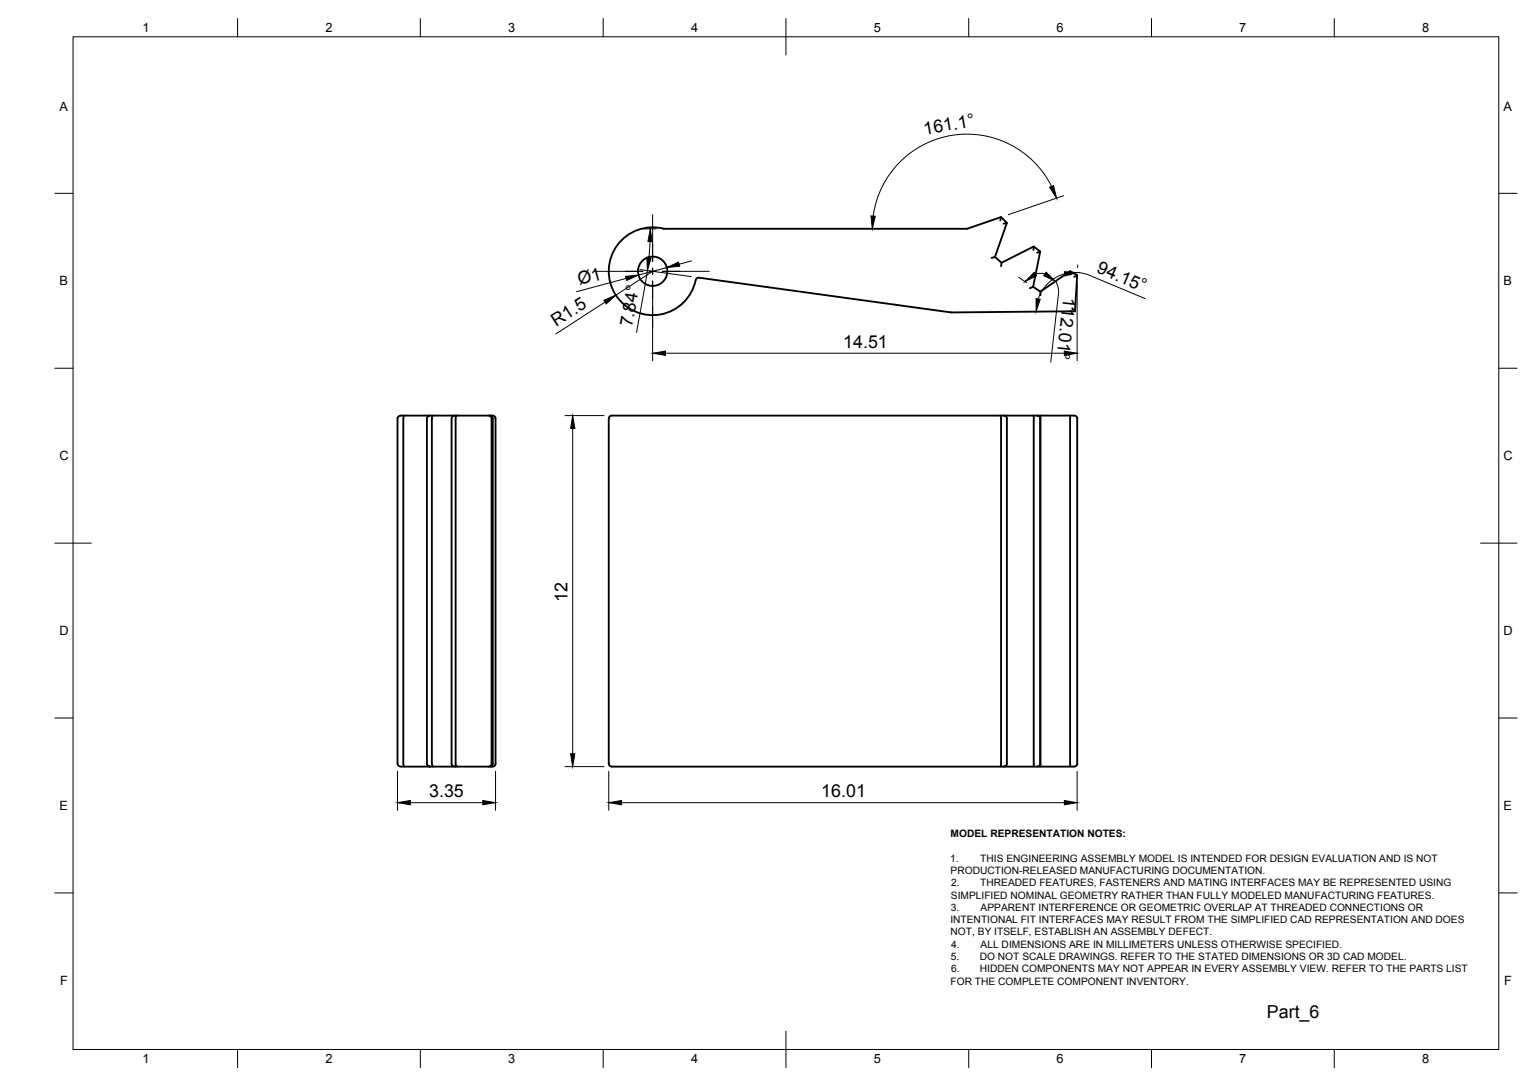
ISO-10303-21;
HEADER;
/* Generated by software containing ST-Developer
 * from STEP Tools, Inc. (www.steptools.com) 
 */

FILE_DESCRIPTION(
/* description */ ('STEP AP242 Edition 2'),
/* implementation_level */ '2;1');

FILE_NAME(
/* name */ 'Part_6.step',
/* time_stamp */ '2026-10-06T10:11:12-07:00',
/* author */ (''),
/* organization */ (''),
/* preprocessor_version */ 'ST-DEVELOPER v20.2',
/* originating_system */ 'Autodesk Translation Framework v15.15.0.0',
/* authorisation */ '');

FILE_SCHEMA (('AUTOMOTIVE_DESIGN { 1 0 10303 214 3 1 1 }'));
ENDSEC;

DATA;
#10=MECHANICAL_DESIGN_GEOMETRIC_PRESENTATION_REPRESENTATION('',(#1793),#54580);
#98=ELLIPSE('',#18957,0.000117970312899575,0.0001);
#99=ELLIPSE('',#18958,0.000120617936713865,0.0001);
#100=ELLIPSE('',#18960,0.000120617936713866,0.0001);
#101=ELLIPSE('',#18962,0.000120617936713866,0.0001);
#102=ELLIPSE('',#18963,0.000120617936713865,0.0001);
#103=ELLIPSE('',#18965,0.000117970312899575,0.0001);
#104=ELLIPSE('',#18967,0.000117970312899575,0.0001);
#105=ELLIPSE('',#18969,0.000117970312899574,0.0001);
#106=ELLIPSE('',#18971,0.000117970312899574,0.0001);
#107=ELLIPSE('',#18973,0.000117970312899575,0.0001);
#108=ELLIPSE('',#18975,0.000120617936713865,0.0001);
#109=ELLIPSE('',#18977,0.000117970312899575,0.0001);
#110=ELLIPSE('',#18979,0.000117970312899575,0.0001);
#111=ELLIPSE('',#18981,0.000120617936713865,0.0001);
#112=ELLIPSE('',#18983,0.000120617936713865,0.0001);
#113=ELLIPSE('',#18985,0.000136567519156022,0.0001);
#114=ELLIPSE('',#18987,0.000136567519156022,0.0001);
#115=ELLIPSE('',#18989,0.000120617936713865,0.0001);
#116=ELLIPSE('',#18991,0.000117970312899574,0.0001);
#117=ELLIPSE('',#19000,0.000117970312899574,0.0001);
#118=ELLIPSE('',#19002,0.000117970312899575,0.0001);
#119=ELLIPSE('',#19008,0.000117970312899575,0.0001);
#149=SPHERICAL_SURFACE('',#19003,0.0001);
#150=SPHERICAL_SURFACE('',#19005,0.0001);
#248=TOROIDAL_SURFACE('',#19023,0.0002,0.0001);
#249=TOROIDAL_SURFACE('',#19025,0.0002,0.0001);
#250=TOROIDAL_SURFACE('',#19027,0.0002,0.0001);
#251=TOROIDAL_SURFACE('',#19029,0.0002,0.0001);
#252=TOROIDAL_SURFACE('',#19033,0.0014,0.0001);
#253=TOROIDAL_SURFACE('',#19035,0.0014,0.0001);
#254=TOROIDAL_SURFACE('',#19039,0.0002,0.0001);
#255=TOROIDAL_SURFACE('',#19041,0.0002,0.0001);
#256=TOROIDAL_SURFACE('',#19044,0.0006,0.0001);
#257=TOROIDAL_SURFACE('',#19046,0.0006,0.0001);
#1749=SHAPE_REPRESENTATION_RELATIONSHIP('SRR','None',#54636,#1763);
#1763=ADVANCED_BREP_SHAPE_REPRESENTATION('',(#1807),#54572);
#1793=STYLED_ITEM('',(#54717),#1807);
#1807=MANIFOLD_SOLID_BREP('Body1',#17672);
#2175=LINE('',#48245,#2768);
#2176=LINE('',#48249,#2769);
#2177=LINE('',#48254,#2770);
#2178=LINE('',#48256,#2771);
#2179=LINE('',#48258,#2772);
#2180=LINE('',#48259,#2773);
#2181=LINE('',#48263,#2774);
#2182=LINE('',#48265,#2775);
#2183=LINE('',#48267,#2776);
#2184=LINE('',#48268,#2777);
#2185=LINE('',#48272,#2778);
#2186=LINE('',#48273,#2779);
#2187=LINE('',#48274,#2780);
#2188=LINE('',#48278,#2781);
#2189=LINE('',#48279,#2782);
#2190=LINE('',#48280,#2783);
#2191=LINE('',#48284,#2784);
#2192=LINE('',#48285,#2785);
#2193=LINE('',#48286,#2786);
#2194=LINE('',#48290,#2787);
#2195=LINE('',#48291,#2788);
#2196=LINE('',#48292,#2789);
#2197=LINE('',#48296,#2790);
#2198=LINE('',#48297,#2791);
#2199=LINE('',#48298,#2792);
#2200=LINE('',#48302,#2793);
#2201=LINE('',#48303,#2794);
#2202=LINE('',#48304,#2795);
#2203=LINE('',#48308,#2796);
#2204=LINE('',#48309,#2797);
#2205=LINE('',#48310,#2798);
#2206=LINE('',#48314,#2799);
#2207=LINE('',#48315,#2800);
#2208=LINE('',#48316,#2801);
#2209=LINE('',#48320,#2802);
#2210=LINE('',#48321,#2803);
#2211=LINE('',#48322,#2804);
#2212=LINE('',#48326,#2805);
#2213=LINE('',#48327,#2806);
#2214=LINE('',#48328,#2807);
#2215=LINE('',#48332,#2808);
#2216=LINE('',#48333,#2809);
#2217=LINE('',#48334,#2810);
#2218=LINE('',#48338,#2811);
#2219=LINE('',#48340,#2812);
#2220=LINE('',#48342,#2813);
#2221=LINE('',#48343,#2814);
#2222=LINE('',#48347,#2815);
#2223=LINE('',#48349,#2816);
#2224=LINE('',#48351,#2817);
#2225=LINE('',#48359,#2818);
#2226=LINE('',#48363,#2819);
#2227=LINE('',#48365,#2820);
#2228=LINE('',#48367,#2821);
#2229=LINE('',#48369,#2822);
#2230=LINE('',#48371,#2823);
#2231=LINE('',#48373,#2824);
#2232=LINE('',#48375,#2825);
#2233=LINE('',#48377,#2826);
#2234=LINE('',#48379,#2827);
#2235=LINE('',#48380,#2828);
#2236=LINE('',#48386,#2829);
#2237=LINE('',#48388,#2830);
#2238=LINE('',#48390,#2831);
#2239=LINE('',#48394,#2832);
#2240=LINE('',#48402,#2833);
#2241=LINE('',#48404,#2834);
#2242=LINE('',#48406,#2835);
#2243=LINE('',#48408,#2836);
#2244=LINE('',#48410,#2837);
#2245=LINE('',#48412,#2838);
#2246=LINE('',#48414,#2839);
#2247=LINE('',#48416,#2840);
#2248=LINE('',#48418,#2841);
#2249=LINE('',#48419,#2842);
#2250=LINE('',#48428,#2843);
#2768=VECTOR('',#22139,1.);
#2769=VECTOR('',#22142,1.);
#2770=VECTOR('',#22147,1.);
#2771=VECTOR('',#22148,1.);
#2772=VECTOR('',#22149,1.);
#2773=VECTOR('',#22150,1.);
#2774=VECTOR('',#22153,1.);
#2775=VECTOR('',#22154,1.);
#2776=VECTOR('',#22155,1.);
#2777=VECTOR('',#22156,1.);
#2778=VECTOR('',#22159,1.);
#2779=VECTOR('',#22160,1.);
#2780=VECTOR('',#22161,1.);
#2781=VECTOR('',#22164,1.);
#2782=VECTOR('',#22165,1.);
#2783=VECTOR('',#22166,1.);
#2784=VECTOR('',#22169,1.);
#2785=VECTOR('',#22170,1.);
#2786=VECTOR('',#22171,1.);
#2787=VECTOR('',#22174,1.);
#2788=VECTOR('',#22175,0.999999999999999);
#2789=VECTOR('',#22176,0.999999999999999);
#2790=VECTOR('',#22179,1.);
#2791=VECTOR('',#22180,1.);
#2792=VECTOR('',#22181,1.);
#2793=VECTOR('',#22184,1.);
#2794=VECTOR('',#22185,1.);
#2795=VECTOR('',#22186,1.);
#2796=VECTOR('',#22189,1.);
#2797=VECTOR('',#22190,1.);
#2798=VECTOR('',#22191,1.);
#2799=VECTOR('',#22194,1.);
#2800=VECTOR('',#22195,1.);
#2801=VECTOR('',#22196,1.);
#2802=VECTOR('',#22199,1.);
#2803=VECTOR('',#22200,1.);
#2804=VECTOR('',#22201,1.);
#2805=VECTOR('',#22204,1.);
#2806=VECTOR('',#22205,1.);
#2807=VECTOR('',#22206,1.);
#2808=VECTOR('',#22209,1.);
#2809=VECTOR('',#22210,1.);
#2810=VECTOR('',#22211,1.);
#2811=VECTOR('',#22214,1.);
#2812=VECTOR('',#22215,1.);
#2813=VECTOR('',#22216,1.);
#2814=VECTOR('',#22217,1.);
#2815=VECTOR('',#22220,1.);
#2816=VECTOR('',#22221,1.);
#2817=VECTOR('',#22222,1.);
#2818=VECTOR('',#22229,1.);
#2819=VECTOR('',#22232,1.);
#2820=VECTOR('',#22233,1.);
#2821=VECTOR('',#22234,1.);
#2822=VECTOR('',#22235,1.);
#2823=VECTOR('',#22236,1.);
#2824=VECTOR('',#22237,1.);
#2825=VECTOR('',#22238,1.);
#2826=VECTOR('',#22239,0.999999999999999);
#2827=VECTOR('',#22240,1.);
#2828=VECTOR('',#22241,1.);
#2829=VECTOR('',#22246,1.);
#2830=VECTOR('',#22247,1.);
#2831=VECTOR('',#22248,1.);
#2832=VECTOR('',#22251,1.);
#2833=VECTOR('',#22258,1.);
#2834=VECTOR('',#22259,1.);
#2835=VECTOR('',#22260,1.);
#2836=VECTOR('',#22261,1.);
#2837=VECTOR('',#22262,1.);
#2838=VECTOR('',#22263,0.999999999999999);
#2839=VECTOR('',#22264,1.);
#2840=VECTOR('',#22265,1.);
#2841=VECTOR('',#22266,1.);
#2842=VECTOR('',#22267,1.);
#2843=VECTOR('',#22276,0.0005);
#3361=CYLINDRICAL_SURFACE('',#18923,0.0015);
#3362=CYLINDRICAL_SURFACE('',#18952,0.0005);
#3363=CYLINDRICAL_SURFACE('',#18956,0.0001);
#3364=CYLINDRICAL_SURFACE('',#18959,0.0001);
#3365=CYLINDRICAL_SURFACE('',#18961,0.0001);
#3366=CYLINDRICAL_SURFACE('',#18964,0.0001);
#3367=CYLINDRICAL_SURFACE('',#18966,0.0001);
#3368=CYLINDRICAL_SURFACE('',#18968,0.0001);
#3369=CYLINDRICAL_SURFACE('',#18970,0.0001);
#3370=CYLINDRICAL_SURFACE('',#18972,0.0001);
#3371=CYLINDRICAL_SURFACE('',#18974,0.0001);
#3372=CYLINDRICAL_SURFACE('',#18976,0.0001);
#3373=CYLINDRICAL_SURFACE('',#18978,0.0001);
#3374=CYLINDRICAL_SURFACE('',#18980,0.0001);
#3375=CYLINDRICAL_SURFACE('',#18982,0.0001);
#3376=CYLINDRICAL_SURFACE('',#18984,0.0001);
#3377=CYLINDRICAL_SURFACE('',#18986,0.0001);
#3378=CYLINDRICAL_SURFACE('',#18988,0.0001);
#3379=CYLINDRICAL_SURFACE('',#18990,0.0001);
#3380=CYLINDRICAL_SURFACE('',#18992,0.0001);
#3381=CYLINDRICAL_SURFACE('',#18994,0.0001);
#3382=CYLINDRICAL_SURFACE('',#18997,0.0001);
#3383=CYLINDRICAL_SURFACE('',#18999,0.0001);
#3384=CYLINDRICAL_SURFACE('',#19001,0.0001);
#3385=CYLINDRICAL_SURFACE('',#19007,0.0001);
#3386=CYLINDRICAL_SURFACE('',#19009,0.0001);
#3387=CYLINDRICAL_SURFACE('',#19011,0.0001);
#3388=CYLINDRICAL_SURFACE('',#19013,0.0001);
#3389=CYLINDRICAL_SURFACE('',#19016,0.0001);
#3390=CYLINDRICAL_SURFACE('',#19018,0.0001);
#3391=CYLINDRICAL_SURFACE('',#19020,0.0001);
#3392=CYLINDRICAL_SURFACE('',#19031,0.0001);
#3393=CYLINDRICAL_SURFACE('',#19037,0.0001);
#3394=CYLINDRICAL_SURFACE('',#19043,0.0001);
#3508=FACE_BOUND('',#5278,.T.);
#3509=FACE_BOUND('',#5280,.T.);
#4225=FACE_OUTER_BOUND('',#5262,.T.);
#4226=FACE_OUTER_BOUND('',#5263,.T.);
#4227=FACE_OUTER_BOUND('',#5264,.T.);
#4228=FACE_OUTER_BOUND('',#5265,.T.);
#4229=FACE_OUTER_BOUND('',#5266,.T.);
#4230=FACE_OUTER_BOUND('',#5267,.T.);
#4231=FACE_OUTER_BOUND('',#5268,.T.);
#4232=FACE_OUTER_BOUND('',#5269,.T.);
#4233=FACE_OUTER_BOUND('',#5270,.T.);
#4234=FACE_OUTER_BOUND('',#5271,.T.);
#4235=FACE_OUTER_BOUND('',#5272,.T.);
#4236=FACE_OUTER_BOUND('',#5273,.T.);
#4237=FACE_OUTER_BOUND('',#5274,.T.);
#4238=FACE_OUTER_BOUND('',#5275,.T.);
#4239=FACE_OUTER_BOUND('',#5276,.T.);
#4240=FACE_OUTER_BOUND('',#5277,.T.);
#4241=FACE_OUTER_BOUND('',#5279,.T.);
#4242=FACE_OUTER_BOUND('',#5281,.T.);
#4243=FACE_OUTER_BOUND('',#5282,.T.);
#4244=FACE_OUTER_BOUND('',#5283,.T.);
#4245=FACE_OUTER_BOUND('',#5284,.T.);
#4246=FACE_OUTER_BOUND('',#5285,.T.);
#4247=FACE_OUTER_BOUND('',#5286,.T.);
#4248=FACE_OUTER_BOUND('',#5287,.T.);
#4249=FACE_OUTER_BOUND('',#5288,.T.);
#4250=FACE_OUTER_BOUND('',#5289,.T.);
#4251=FACE_OUTER_BOUND('',#5290,.T.);
#4252=FACE_OUTER_BOUND('',#5291,.T.);
#4253=FACE_OUTER_BOUND('',#5292,.T.);
#4254=FACE_OUTER_BOUND('',#5293,.T.);
#4255=FACE_OUTER_BOUND('',#5294,.T.);
#4256=FACE_OUTER_BOUND('',#5295,.T.);
#4257=FACE_OUTER_BOUND('',#5296,.T.);
#4258=FACE_OUTER_BOUND('',#5297,.T.);
#4259=FACE_OUTER_BOUND('',#5298,.T.);
#4260=FACE_OUTER_BOUND('',#5299,.T.);
#4261=FACE_OUTER_BOUND('',#5300,.T.);
#4262=FACE_OUTER_BOUND('',#5301,.T.);
#4263=FACE_OUTER_BOUND('',#5302,.T.);
#4264=FACE_OUTER_BOUND('',#5303,.T.);
#4265=FACE_OUTER_BOUND('',#5304,.T.);
#4266=FACE_OUTER_BOUND('',#5305,.T.);
#4267=FACE_OUTER_BOUND('',#5306,.T.);
#4268=FACE_OUTER_BOUND('',#5307,.T.);
#4269=FACE_OUTER_BOUND('',#5308,.T.);
#4270=FACE_OUTER_BOUND('',#5309,.T.);
#4271=FACE_OUTER_BOUND('',#5310,.T.);
#4272=FACE_OUTER_BOUND('',#5311,.T.);
#4273=FACE_OUTER_BOUND('',#5312,.T.);
#4274=FACE_OUTER_BOUND('',#5313,.T.);
#4275=FACE_OUTER_BOUND('',#5314,.T.);
#4276=FACE_OUTER_BOUND('',#5315,.T.);
#4277=FACE_OUTER_BOUND('',#5316,.T.);
#4278=FACE_OUTER_BOUND('',#5317,.T.);
#4279=FACE_OUTER_BOUND('',#5318,.T.);
#4280=FACE_OUTER_BOUND('',#5319,.T.);
#4281=FACE_OUTER_BOUND('',#5320,.T.);
#4282=FACE_OUTER_BOUND('',#5321,.T.);
#4283=FACE_OUTER_BOUND('',#5322,.T.);
#4284=FACE_OUTER_BOUND('',#5323,.T.);
#4285=FACE_OUTER_BOUND('',#5324,.T.);
#4286=FACE_OUTER_BOUND('',#5325,.T.);
#5262=EDGE_LOOP('',(#14995,#14996,#14997,#14998));
#5263=EDGE_LOOP('',(#14999,#15000,#15001,#15002));
#5264=EDGE_LOOP('',(#15003,#15004,#15005,#15006));
#5265=EDGE_LOOP('',(#15007,#15008,#15009,#15010));
#5266=EDGE_LOOP('',(#15011,#15012,#15013,#15014));
#5267=EDGE_LOOP('',(#15015,#15016,#15017,#15018));
#5268=EDGE_LOOP('',(#15019,#15020,#15021,#15022));
#5269=EDGE_LOOP('',(#15023,#15024,#15025,#15026));
#5270=EDGE_LOOP('',(#15027,#15028,#15029,#15030));
#5271=EDGE_LOOP('',(#15031,#15032,#15033,#15034));
#5272=EDGE_LOOP('',(#15035,#15036,#15037,#15038));
#5273=EDGE_LOOP('',(#15039,#15040,#15041,#15042));
#5274=EDGE_LOOP('',(#15043,#15044,#15045,#15046));
#5275=EDGE_LOOP('',(#15047,#15048,#15049,#15050));
#5276=EDGE_LOOP('',(#15051,#15052,#15053,#15054));
#5277=EDGE_LOOP('',(#15055,#15056,#15057,#15058,#15059,#15060,#15061,#15062,
#15063,#15064,#15065,#15066,#15067,#15068,#15069,#15070,#15071,#15072));
#5278=EDGE_LOOP('',(#15073));
#5279=EDGE_LOOP('',(#15074,#15075,#15076,#15077,#15078,#15079,#15080,#15081,
#15082,#15083,#15084,#15085,#15086,#15087,#15088,#15089,#15090,#15091));
#5280=EDGE_LOOP('',(#15092));
#5281=EDGE_LOOP('',(#15093,#15094,#15095,#15096,#15097));
#5282=EDGE_LOOP('',(#15098,#15099,#15100,#15101));
#5283=EDGE_LOOP('',(#15102,#15103,#15104,#15105));
#5284=EDGE_LOOP('',(#15106,#15107,#15108,#15109));
#5285=EDGE_LOOP('',(#15110,#15111,#15112,#15113));
#5286=EDGE_LOOP('',(#15114,#15115,#15116,#15117));
#5287=EDGE_LOOP('',(#15118,#15119,#15120,#15121));
#5288=EDGE_LOOP('',(#15122,#15123,#15124,#15125));
#5289=EDGE_LOOP('',(#15126,#15127,#15128,#15129));
#5290=EDGE_LOOP('',(#15130,#15131,#15132,#15133));
#5291=EDGE_LOOP('',(#15134,#15135,#15136,#15137));
#5292=EDGE_LOOP('',(#15138,#15139,#15140,#15141));
#5293=EDGE_LOOP('',(#15142,#15143,#15144,#15145));
#5294=EDGE_LOOP('',(#15146,#15147,#15148,#15149));
#5295=EDGE_LOOP('',(#15150,#15151,#15152,#15153));
#5296=EDGE_LOOP('',(#15154,#15155,#15156,#15157));
#5297=EDGE_LOOP('',(#15158,#15159,#15160,#15161));
#5298=EDGE_LOOP('',(#15162,#15163,#15164,#15165));
#5299=EDGE_LOOP('',(#15166,#15167,#15168,#15169));
#5300=EDGE_LOOP('',(#15170,#15171,#15172,#15173));
#5301=EDGE_LOOP('',(#15174,#15175,#15176,#15177));
#5302=EDGE_LOOP('',(#15178,#15179,#15180,#15181));
#5303=EDGE_LOOP('',(#15182,#15183,#15184,#15185));
#5304=EDGE_LOOP('',(#15186,#15187,#15188));
#5305=EDGE_LOOP('',(#15189,#15190,#15191));
#5306=EDGE_LOOP('',(#15192,#15193,#15194,#15195));
#5307=EDGE_LOOP('',(#15196,#15197,#15198,#15199));
#5308=EDGE_LOOP('',(#15200,#15201,#15202,#15203));
#5309=EDGE_LOOP('',(#15204,#15205,#15206,#15207));
#5310=EDGE_LOOP('',(#15208,#15209,#15210,#15211));
#5311=EDGE_LOOP('',(#15212,#15213,#15214,#15215));
#5312=EDGE_LOOP('',(#15216,#15217,#15218,#15219));
#5313=EDGE_LOOP('',(#15220,#15221,#15222,#15223));
#5314=EDGE_LOOP('',(#15224,#15225,#15226,#15227));
#5315=EDGE_LOOP('',(#15228,#15229,#15230,#15231));
#5316=EDGE_LOOP('',(#15232,#15233,#15234,#15235));
#5317=EDGE_LOOP('',(#15236,#15237,#15238,#15239));
#5318=EDGE_LOOP('',(#15240,#15241,#15242,#15243));
#5319=EDGE_LOOP('',(#15244,#15245,#15246,#15247));
#5320=EDGE_LOOP('',(#15248,#15249,#15250,#15251));
#5321=EDGE_LOOP('',(#15252,#15253,#15254,#15255));
#5322=EDGE_LOOP('',(#15256,#15257,#15258,#15259));
#5323=EDGE_LOOP('',(#15260,#15261,#15262,#15263));
#5324=EDGE_LOOP('',(#15264,#15265,#15266,#15267));
#5325=EDGE_LOOP('',(#15268,#15269,#15270,#15271,#15272));
#6186=CIRCLE('',#18924,0.0015);
#6187=CIRCLE('',#18925,0.0015);
#6188=CIRCLE('',#18941,0.0002);
#6189=CIRCLE('',#18942,0.0014);
#6190=CIRCLE('',#18943,0.0002);
#6191=CIRCLE('',#18944,0.0002);
#6192=CIRCLE('',#18945,0.0006);
#6193=CIRCLE('',#18947,0.0002);
#6194=CIRCLE('',#18948,0.0002);
#6195=CIRCLE('',#18949,0.0014);
#6196=CIRCLE('',#18950,0.0002);
#6197=CIRCLE('',#18951,0.0006);
#6198=CIRCLE('',#18953,0.0005);
#6199=CIRCLE('',#18954,0.0005);
#6200=CIRCLE('',#18955,0.0005);
#6201=CIRCLE('',#18993,0.0001);
#6202=CIRCLE('',#18995,0.0001);
#6203=CIRCLE('',#18996,0.0001);
#6204=CIRCLE('',#18998,0.0001);
#6205=CIRCLE('',#19004,0.0001);
#6206=CIRCLE('',#19006,0.0001);
#6207=CIRCLE('',#19010,0.0001);
#6208=CIRCLE('',#19012,0.0001);
#6209=CIRCLE('',#19014,0.0001);
#6210=CIRCLE('',#19015,0.0001);
#6211=CIRCLE('',#19017,0.0001);
#6212=CIRCLE('',#19019,0.0001);
#6213=CIRCLE('',#19021,0.0001);
#6214=CIRCLE('',#19022,0.0001);
#6215=CIRCLE('',#19024,0.0001);
#6216=CIRCLE('',#19026,0.0001);
#6217=CIRCLE('',#19028,0.0001);
#6218=CIRCLE('',#19030,0.0001);
#6219=CIRCLE('',#19032,0.0001);
#6220=CIRCLE('',#19034,0.0001);
#6221=CIRCLE('',#19036,0.0001);
#6222=CIRCLE('',#19038,0.0001);
#6223=CIRCLE('',#19040,0.0001);
#6224=CIRCLE('',#19042,0.0001);
#6225=CIRCLE('',#19045,0.0001);
#6226=CIRCLE('',#19047,0.0001);
#7845=VERTEX_POINT('',#48243);
#7846=VERTEX_POINT('',#48244);
#7847=VERTEX_POINT('',#48246);
#7848=VERTEX_POINT('',#48248);
#7849=VERTEX_POINT('',#48252);
#7850=VERTEX_POINT('',#48253);
#7851=VERTEX_POINT('',#48255);
#7852=VERTEX_POINT('',#48257);
#7853=VERTEX_POINT('',#48261);
#7854=VERTEX_POINT('',#48262);
#7855=VERTEX_POINT('',#48264);
#7856=VERTEX_POINT('',#48266);
#7857=VERTEX_POINT('',#48270);
#7858=VERTEX_POINT('',#48271);
#7859=VERTEX_POINT('',#48276);
#7860=VERTEX_POINT('',#48277);
#7861=VERTEX_POINT('',#48282);
#7862=VERTEX_POINT('',#48283);
#7863=VERTEX_POINT('',#48288);
#7864=VERTEX_POINT('',#48289);
#7865=VERTEX_POINT('',#48294);
#7866=VERTEX_POINT('',#48295);
#7867=VERTEX_POINT('',#48300);
#7868=VERTEX_POINT('',#48301);
#7869=VERTEX_POINT('',#48306);
#7870=VERTEX_POINT('',#48307);
#7871=VERTEX_POINT('',#48312);
#7872=VERTEX_POINT('',#48313);
#7873=VERTEX_POINT('',#48318);
#7874=VERTEX_POINT('',#48319);
#7875=VERTEX_POINT('',#48324);
#7876=VERTEX_POINT('',#48325);
#7877=VERTEX_POINT('',#48330);
#7878=VERTEX_POINT('',#48331);
#7879=VERTEX_POINT('',#48336);
#7880=VERTEX_POINT('',#48337);
#7881=VERTEX_POINT('',#48339);
#7882=VERTEX_POINT('',#48341);
#7883=VERTEX_POINT('',#48345);
#7884=VERTEX_POINT('',#48346);
#7885=VERTEX_POINT('',#48348);
#7886=VERTEX_POINT('',#48350);
#7887=VERTEX_POINT('',#48352);
#7888=VERTEX_POINT('',#48354);
#7889=VERTEX_POINT('',#48356);
#7890=VERTEX_POINT('',#48358);
#7891=VERTEX_POINT('',#48360);
#7892=VERTEX_POINT('',#48362);
#7893=VERTEX_POINT('',#48364);
#7894=VERTEX_POINT('',#48366);
#7895=VERTEX_POINT('',#48368);
#7896=VERTEX_POINT('',#48370);
#7897=VERTEX_POINT('',#48372);
#7898=VERTEX_POINT('',#48374);
#7899=VERTEX_POINT('',#48376);
#7900=VERTEX_POINT('',#48378);
#7901=VERTEX_POINT('',#48381);
#7902=VERTEX_POINT('',#48384);
#7903=VERTEX_POINT('',#48385);
#7904=VERTEX_POINT('',#48387);
#7905=VERTEX_POINT('',#48389);
#7906=VERTEX_POINT('',#48391);
#7907=VERTEX_POINT('',#48393);
#7908=VERTEX_POINT('',#48395);
#7909=VERTEX_POINT('',#48397);
#7910=VERTEX_POINT('',#48399);
#7911=VERTEX_POINT('',#48401);
#7912=VERTEX_POINT('',#48403);
#7913=VERTEX_POINT('',#48405);
#7914=VERTEX_POINT('',#48407);
#7915=VERTEX_POINT('',#48409);
#7916=VERTEX_POINT('',#48411);
#7917=VERTEX_POINT('',#48413);
#7918=VERTEX_POINT('',#48415);
#7919=VERTEX_POINT('',#48417);
#7920=VERTEX_POINT('',#48420);
#7921=VERTEX_POINT('',#48423);
#7922=VERTEX_POINT('',#48424);
#7923=VERTEX_POINT('',#48427);
#10289=EDGE_CURVE('',#7845,#7846,#2175,.F.);
#10290=EDGE_CURVE('',#7846,#7847,#6186,.F.);
#10291=EDGE_CURVE('',#7847,#7848,#2176,.T.);
#10292=EDGE_CURVE('',#7848,#7845,#6187,.F.);
#10293=EDGE_CURVE('',#7849,#7850,#2177,.F.);
#10294=EDGE_CURVE('',#7850,#7851,#2178,.F.);
#10295=EDGE_CURVE('',#7851,#7852,#2179,.F.);
#10296=EDGE_CURVE('',#7852,#7849,#2180,.T.);
#10297=EDGE_CURVE('',#7853,#7854,#2181,.T.);
#10298=EDGE_CURVE('',#7853,#7855,#2182,.F.);
#10299=EDGE_CURVE('',#7855,#7856,#2183,.T.);
#10300=EDGE_CURVE('',#7856,#7854,#2184,.T.);
#10301=EDGE_CURVE('',#7857,#7858,#2185,.T.);
#10302=EDGE_CURVE('',#7857,#7853,#2186,.F.);
#10303=EDGE_CURVE('',#7854,#7858,#2187,.T.);
#10304=EDGE_CURVE('',#7859,#7860,#2188,.T.);
#10305=EDGE_CURVE('',#7859,#7857,#2189,.F.);
#10306=EDGE_CURVE('',#7858,#7860,#2190,.T.);
#10307=EDGE_CURVE('',#7861,#7862,#2191,.T.);
#10308=EDGE_CURVE('',#7861,#7859,#2192,.F.);
#10309=EDGE_CURVE('',#7860,#7862,#2193,.T.);
#10310=EDGE_CURVE('',#7863,#7864,#2194,.T.);
#10311=EDGE_CURVE('',#7863,#7861,#2195,.F.);
#10312=EDGE_CURVE('',#7862,#7864,#2196,.T.);
#10313=EDGE_CURVE('',#7865,#7866,#2197,.T.);
#10314=EDGE_CURVE('',#7865,#7863,#2198,.F.);
#10315=EDGE_CURVE('',#7864,#7866,#2199,.T.);
#10316=EDGE_CURVE('',#7867,#7868,#2200,.T.);
#10317=EDGE_CURVE('',#7867,#7865,#2201,.F.);
#10318=EDGE_CURVE('',#7866,#7868,#2202,.T.);
#10319=EDGE_CURVE('',#7869,#7870,#2203,.T.);
#10320=EDGE_CURVE('',#7869,#7867,#2204,.F.);
#10321=EDGE_CURVE('',#7868,#7870,#2205,.T.);
#10322=EDGE_CURVE('',#7871,#7872,#2206,.T.);
#10323=EDGE_CURVE('',#7871,#7869,#2207,.F.);
#10324=EDGE_CURVE('',#7870,#7872,#2208,.T.);
#10325=EDGE_CURVE('',#7873,#7874,#2209,.T.);
#10326=EDGE_CURVE('',#7873,#7871,#2210,.F.);
#10327=EDGE_CURVE('',#7872,#7874,#2211,.T.);
#10328=EDGE_CURVE('',#7875,#7876,#2212,.T.);
#10329=EDGE_CURVE('',#7875,#7873,#2213,.F.);
#10330=EDGE_CURVE('',#7874,#7876,#2214,.T.);
#10331=EDGE_CURVE('',#7877,#7878,#2215,.F.);
#10332=EDGE_CURVE('',#7878,#7875,#2216,.F.);
#10333=EDGE_CURVE('',#7876,#7877,#2217,.T.);
#10334=EDGE_CURVE('',#7879,#7880,#2218,.T.);
#10335=EDGE_CURVE('',#7880,#7881,#2219,.F.);
#10336=EDGE_CURVE('',#7881,#7882,#2220,.T.);
#10337=EDGE_CURVE('',#7882,#7879,#2221,.T.);
#10338=EDGE_CURVE('',#7883,#7884,#2222,.F.);
#10339=EDGE_CURVE('',#7884,#7885,#2223,.F.);
#10340=EDGE_CURVE('',#7885,#7886,#2224,.F.);
#10341=EDGE_CURVE('',#7887,#7886,#6188,.T.);
#10342=EDGE_CURVE('',#7887,#7888,#6189,.T.);
#10343=EDGE_CURVE('',#7889,#7888,#6190,.T.);
#10344=EDGE_CURVE('',#7889,#7890,#2225,.F.);
#10345=EDGE_CURVE('',#7891,#7890,#6191,.T.);
#10346=EDGE_CURVE('',#7891,#7892,#2226,.F.);
#10347=EDGE_CURVE('',#7892,#7893,#2227,.F.);
#10348=EDGE_CURVE('',#7893,#7894,#2228,.F.);
#10349=EDGE_CURVE('',#7894,#7895,#2229,.F.);
#10350=EDGE_CURVE('',#7895,#7896,#2230,.F.);
#10351=EDGE_CURVE('',#7896,#7897,#2231,.F.);
#10352=EDGE_CURVE('',#7897,#7898,#2232,.F.);
#10353=EDGE_CURVE('',#7898,#7899,#2233,.F.);
#10354=EDGE_CURVE('',#7899,#7900,#2234,.F.);
#10355=EDGE_CURVE('',#7900,#7883,#2235,.F.);
#10356=EDGE_CURVE('',#7901,#7901,#6192,.F.);
#10357=EDGE_CURVE('',#7902,#7903,#2236,.T.);
#10358=EDGE_CURVE('',#7903,#7904,#2237,.T.);
#10359=EDGE_CURVE('',#7904,#7905,#2238,.T.);
#10360=EDGE_CURVE('',#7906,#7905,#6193,.T.);
#10361=EDGE_CURVE('',#7906,#7907,#2239,.T.);
#10362=EDGE_CURVE('',#7908,#7907,#6194,.T.);
#10363=EDGE_CURVE('',#7908,#7909,#6195,.T.);
#10364=EDGE_CURVE('',#7910,#7909,#6196,.T.);
#10365=EDGE_CURVE('',#7910,#7911,#2240,.T.);
#10366=EDGE_CURVE('',#7911,#7912,#2241,.T.);
#10367=EDGE_CURVE('',#7912,#7913,#2242,.T.);
#10368=EDGE_CURVE('',#7913,#7914,#2243,.T.);
#10369=EDGE_CURVE('',#7914,#7915,#2244,.T.);
#10370=EDGE_CURVE('',#7915,#7916,#2245,.T.);
#10371=EDGE_CURVE('',#7916,#7917,#2246,.T.);
#10372=EDGE_CURVE('',#7917,#7918,#2247,.T.);
#10373=EDGE_CURVE('',#7918,#7919,#2248,.T.);
#10374=EDGE_CURVE('',#7919,#7902,#2249,.T.);
#10375=EDGE_CURVE('',#7920,#7920,#6197,.F.);
#10376=EDGE_CURVE('',#7921,#7922,#6198,.T.);
#10377=EDGE_CURVE('',#7922,#7921,#6199,.T.);
#10378=EDGE_CURVE('',#7921,#7923,#2250,.T.);
#10379=EDGE_CURVE('',#7923,#7923,#6200,.T.);
#10380=EDGE_CURVE('',#7917,#7865,#98,.F.);
#10381=EDGE_CURVE('',#7863,#7916,#99,.T.);
#10382=EDGE_CURVE('',#7861,#7915,#100,.T.);
#10383=EDGE_CURVE('',#7899,#7862,#101,.T.);
#10384=EDGE_CURVE('',#7864,#7898,#102,.F.);
#10385=EDGE_CURVE('',#7866,#7897,#103,.F.);
#10386=EDGE_CURVE('',#7918,#7867,#104,.F.);
#10387=EDGE_CURVE('',#7859,#7914,#105,.T.);
#10388=EDGE_CURVE('',#7900,#7860,#106,.T.);
#10389=EDGE_CURVE('',#7868,#7896,#107,.F.);
#10390=EDGE_CURVE('',#7919,#7869,#108,.F.);
#10391=EDGE_CURVE('',#7857,#7913,#109,.T.);
#10392=EDGE_CURVE('',#7883,#7858,#110,.T.);
#10393=EDGE_CURVE('',#7870,#7895,#111,.F.);
#10394=EDGE_CURVE('',#7902,#7871,#112,.F.);
#10395=EDGE_CURVE('',#7853,#7912,#113,.T.);
#10396=EDGE_CURVE('',#7884,#7854,#114,.T.);
#10397=EDGE_CURVE('',#7872,#7894,#115,.F.);
#10398=EDGE_CURVE('',#7903,#7873,#116,.F.);
#10399=EDGE_CURVE('',#7855,#7911,#6201,.T.);
#10400=EDGE_CURVE('',#7856,#7849,#6202,.T.);
#10401=EDGE_CURVE('',#7850,#7855,#6203,.T.);
#10402=EDGE_CURVE('',#7885,#7856,#6204,.T.);
#10403=EDGE_CURVE('',#7874,#7893,#117,.F.);
#10404=EDGE_CURVE('',#7904,#7875,#118,.F.);
#10405=EDGE_CURVE('',#7850,#7911,#6205,.F.);
#10406=EDGE_CURVE('',#7885,#7849,#6206,.F.);
#10407=EDGE_CURVE('',#7876,#7892,#119,.F.);
#10408=EDGE_CURVE('',#7905,#7878,#6207,.T.);
#10409=EDGE_CURVE('',#7851,#7910,#6208,.T.);
#10410=EDGE_CURVE('',#7852,#7845,#6209,.F.);
#10411=EDGE_CURVE('',#7846,#7851,#6210,.F.);
#10412=EDGE_CURVE('',#7886,#7852,#6211,.T.);
#10413=EDGE_CURVE('',#7877,#7891,#6212,.T.);
#10414=EDGE_CURVE('',#7878,#7881,#6213,.F.);
#10415=EDGE_CURVE('',#7882,#7877,#6214,.F.);
#10416=EDGE_CURVE('',#7906,#7881,#6215,.F.);
#10417=EDGE_CURVE('',#7846,#7909,#6216,.F.);
#10418=EDGE_CURVE('',#7887,#7845,#6217,.F.);
#10419=EDGE_CURVE('',#7882,#7890,#6218,.F.);
#10420=EDGE_CURVE('',#7907,#7880,#6219,.T.);
#10421=EDGE_CURVE('',#7847,#7908,#6220,.T.);
#10422=EDGE_CURVE('',#7888,#7848,#6221,.T.);
#10423=EDGE_CURVE('',#7879,#7889,#6222,.T.);
#10424=EDGE_CURVE('',#7847,#7880,#6223,.T.);
#10425=EDGE_CURVE('',#7879,#7848,#6224,.T.);
#10426=EDGE_CURVE('',#7923,#7920,#6225,.T.);
#10427=EDGE_CURVE('',#7922,#7901,#6226,.T.);
#14995=ORIENTED_EDGE('',*,*,#10289,.T.);
#14996=ORIENTED_EDGE('',*,*,#10290,.T.);
#14997=ORIENTED_EDGE('',*,*,#10291,.T.);
#14998=ORIENTED_EDGE('',*,*,#10292,.T.);
#14999=ORIENTED_EDGE('',*,*,#10293,.T.);
#15000=ORIENTED_EDGE('',*,*,#10294,.T.);
#15001=ORIENTED_EDGE('',*,*,#10295,.T.);
#15002=ORIENTED_EDGE('',*,*,#10296,.T.);
#15003=ORIENTED_EDGE('',*,*,#10297,.F.);
#15004=ORIENTED_EDGE('',*,*,#10298,.T.);
#15005=ORIENTED_EDGE('',*,*,#10299,.T.);
#15006=ORIENTED_EDGE('',*,*,#10300,.T.);
#15007=ORIENTED_EDGE('',*,*,#10301,.F.);
#15008=ORIENTED_EDGE('',*,*,#10302,.T.);
#15009=ORIENTED_EDGE('',*,*,#10297,.T.);
#15010=ORIENTED_EDGE('',*,*,#10303,.T.);
#15011=ORIENTED_EDGE('',*,*,#10304,.F.);
#15012=ORIENTED_EDGE('',*,*,#10305,.T.);
#15013=ORIENTED_EDGE('',*,*,#10301,.T.);
#15014=ORIENTED_EDGE('',*,*,#10306,.T.);
#15015=ORIENTED_EDGE('',*,*,#10307,.F.);
#15016=ORIENTED_EDGE('',*,*,#10308,.T.);
#15017=ORIENTED_EDGE('',*,*,#10304,.T.);
#15018=ORIENTED_EDGE('',*,*,#10309,.T.);
#15019=ORIENTED_EDGE('',*,*,#10310,.F.);
#15020=ORIENTED_EDGE('',*,*,#10311,.T.);
#15021=ORIENTED_EDGE('',*,*,#10307,.T.);
#15022=ORIENTED_EDGE('',*,*,#10312,.T.);
#15023=ORIENTED_EDGE('',*,*,#10313,.F.);
#15024=ORIENTED_EDGE('',*,*,#10314,.T.);
#15025=ORIENTED_EDGE('',*,*,#10310,.T.);
#15026=ORIENTED_EDGE('',*,*,#10315,.T.);
#15027=ORIENTED_EDGE('',*,*,#10316,.F.);
#15028=ORIENTED_EDGE('',*,*,#10317,.T.);
#15029=ORIENTED_EDGE('',*,*,#10313,.T.);
#15030=ORIENTED_EDGE('',*,*,#10318,.T.);
#15031=ORIENTED_EDGE('',*,*,#10319,.F.);
#15032=ORIENTED_EDGE('',*,*,#10320,.T.);
#15033=ORIENTED_EDGE('',*,*,#10316,.T.);
#15034=ORIENTED_EDGE('',*,*,#10321,.T.);
#15035=ORIENTED_EDGE('',*,*,#10322,.F.);
#15036=ORIENTED_EDGE('',*,*,#10323,.T.);
#15037=ORIENTED_EDGE('',*,*,#10319,.T.);
#15038=ORIENTED_EDGE('',*,*,#10324,.T.);
#15039=ORIENTED_EDGE('',*,*,#10325,.F.);
#15040=ORIENTED_EDGE('',*,*,#10326,.T.);
#15041=ORIENTED_EDGE('',*,*,#10322,.T.);
#15042=ORIENTED_EDGE('',*,*,#10327,.T.);
#15043=ORIENTED_EDGE('',*,*,#10328,.F.);
#15044=ORIENTED_EDGE('',*,*,#10329,.T.);
#15045=ORIENTED_EDGE('',*,*,#10325,.T.);
#15046=ORIENTED_EDGE('',*,*,#10330,.T.);
#15047=ORIENTED_EDGE('',*,*,#10331,.T.);
#15048=ORIENTED_EDGE('',*,*,#10332,.T.);
#15049=ORIENTED_EDGE('',*,*,#10328,.T.);
#15050=ORIENTED_EDGE('',*,*,#10333,.T.);
#15051=ORIENTED_EDGE('',*,*,#10334,.T.);
#15052=ORIENTED_EDGE('',*,*,#10335,.T.);
#15053=ORIENTED_EDGE('',*,*,#10336,.T.);
#15054=ORIENTED_EDGE('',*,*,#10337,.T.);
#15055=ORIENTED_EDGE('',*,*,#10338,.T.);
#15056=ORIENTED_EDGE('',*,*,#10339,.T.);
#15057=ORIENTED_EDGE('',*,*,#10340,.T.);
#15058=ORIENTED_EDGE('',*,*,#10341,.F.);
#15059=ORIENTED_EDGE('',*,*,#10342,.T.);
#15060=ORIENTED_EDGE('',*,*,#10343,.F.);
#15061=ORIENTED_EDGE('',*,*,#10344,.T.);
#15062=ORIENTED_EDGE('',*,*,#10345,.F.);
#15063=ORIENTED_EDGE('',*,*,#10346,.T.);
#15064=ORIENTED_EDGE('',*,*,#10347,.T.);
#15065=ORIENTED_EDGE('',*,*,#10348,.T.);
#15066=ORIENTED_EDGE('',*,*,#10349,.T.);
#15067=ORIENTED_EDGE('',*,*,#10350,.T.);
#15068=ORIENTED_EDGE('',*,*,#10351,.T.);
#15069=ORIENTED_EDGE('',*,*,#10352,.T.);
#15070=ORIENTED_EDGE('',*,*,#10353,.T.);
#15071=ORIENTED_EDGE('',*,*,#10354,.T.);
#15072=ORIENTED_EDGE('',*,*,#10355,.T.);
#15073=ORIENTED_EDGE('',*,*,#10356,.T.);
#15074=ORIENTED_EDGE('',*,*,#10357,.T.);
#15075=ORIENTED_EDGE('',*,*,#10358,.T.);
#15076=ORIENTED_EDGE('',*,*,#10359,.T.);
#15077=ORIENTED_EDGE('',*,*,#10360,.F.);
#15078=ORIENTED_EDGE('',*,*,#10361,.T.);
#15079=ORIENTED_EDGE('',*,*,#10362,.F.);
#15080=ORIENTED_EDGE('',*,*,#10363,.T.);
#15081=ORIENTED_EDGE('',*,*,#10364,.F.);
#15082=ORIENTED_EDGE('',*,*,#10365,.T.);
#15083=ORIENTED_EDGE('',*,*,#10366,.T.);
#15084=ORIENTED_EDGE('',*,*,#10367,.T.);
#15085=ORIENTED_EDGE('',*,*,#10368,.T.);
#15086=ORIENTED_EDGE('',*,*,#10369,.T.);
#15087=ORIENTED_EDGE('',*,*,#10370,.T.);
#15088=ORIENTED_EDGE('',*,*,#10371,.T.);
#15089=ORIENTED_EDGE('',*,*,#10372,.T.);
#15090=ORIENTED_EDGE('',*,*,#10373,.T.);
#15091=ORIENTED_EDGE('',*,*,#10374,.T.);
#15092=ORIENTED_EDGE('',*,*,#10375,.T.);
#15093=ORIENTED_EDGE('',*,*,#10376,.T.);
#15094=ORIENTED_EDGE('',*,*,#10377,.T.);
#15095=ORIENTED_EDGE('',*,*,#10378,.T.);
#15096=ORIENTED_EDGE('',*,*,#10379,.T.);
#15097=ORIENTED_EDGE('',*,*,#10378,.F.);
#15098=ORIENTED_EDGE('',*,*,#10380,.F.);
#15099=ORIENTED_EDGE('',*,*,#10371,.F.);
#15100=ORIENTED_EDGE('',*,*,#10381,.F.);
#15101=ORIENTED_EDGE('',*,*,#10314,.F.);
#15102=ORIENTED_EDGE('',*,*,#10381,.T.);
#15103=ORIENTED_EDGE('',*,*,#10370,.F.);
#15104=ORIENTED_EDGE('',*,*,#10382,.F.);
#15105=ORIENTED_EDGE('',*,*,#10311,.F.);
#15106=ORIENTED_EDGE('',*,*,#10383,.F.);
#15107=ORIENTED_EDGE('',*,*,#10353,.F.);
#15108=ORIENTED_EDGE('',*,*,#10384,.F.);
#15109=ORIENTED_EDGE('',*,*,#10312,.F.);
#15110=ORIENTED_EDGE('',*,*,#10384,.T.);
#15111=ORIENTED_EDGE('',*,*,#10352,.F.);
#15112=ORIENTED_EDGE('',*,*,#10385,.F.);
#15113=ORIENTED_EDGE('',*,*,#10315,.F.);
#15114=ORIENTED_EDGE('',*,*,#10380,.T.);
#15115=ORIENTED_EDGE('',*,*,#10317,.F.);
#15116=ORIENTED_EDGE('',*,*,#10386,.F.);
#15117=ORIENTED_EDGE('',*,*,#10372,.F.);
#15118=ORIENTED_EDGE('',*,*,#10382,.T.);
#15119=ORIENTED_EDGE('',*,*,#10369,.F.);
#15120=ORIENTED_EDGE('',*,*,#10387,.F.);
#15121=ORIENTED_EDGE('',*,*,#10308,.F.);
#15122=ORIENTED_EDGE('',*,*,#10383,.T.);
#15123=ORIENTED_EDGE('',*,*,#10309,.F.);
#15124=ORIENTED_EDGE('',*,*,#10388,.F.);
#15125=ORIENTED_EDGE('',*,*,#10354,.F.);
#15126=ORIENTED_EDGE('',*,*,#10385,.T.);
#15127=ORIENTED_EDGE('',*,*,#10351,.F.);
#15128=ORIENTED_EDGE('',*,*,#10389,.F.);
#15129=ORIENTED_EDGE('',*,*,#10318,.F.);
#15130=ORIENTED_EDGE('',*,*,#10386,.T.);
#15131=ORIENTED_EDGE('',*,*,#10320,.F.);
#15132=ORIENTED_EDGE('',*,*,#10390,.F.);
#15133=ORIENTED_EDGE('',*,*,#10373,.F.);
#15134=ORIENTED_EDGE('',*,*,#10387,.T.);
#15135=ORIENTED_EDGE('',*,*,#10368,.F.);
#15136=ORIENTED_EDGE('',*,*,#10391,.F.);
#15137=ORIENTED_EDGE('',*,*,#10305,.F.);
#15138=ORIENTED_EDGE('',*,*,#10388,.T.);
#15139=ORIENTED_EDGE('',*,*,#10306,.F.);
#15140=ORIENTED_EDGE('',*,*,#10392,.F.);
#15141=ORIENTED_EDGE('',*,*,#10355,.F.);
#15142=ORIENTED_EDGE('',*,*,#10389,.T.);
#15143=ORIENTED_EDGE('',*,*,#10350,.F.);
#15144=ORIENTED_EDGE('',*,*,#10393,.F.);
#15145=ORIENTED_EDGE('',*,*,#10321,.F.);
#15146=ORIENTED_EDGE('',*,*,#10390,.T.);
#15147=ORIENTED_EDGE('',*,*,#10323,.F.);
#15148=ORIENTED_EDGE('',*,*,#10394,.F.);
#15149=ORIENTED_EDGE('',*,*,#10374,.F.);
#15150=ORIENTED_EDGE('',*,*,#10391,.T.);
#15151=ORIENTED_EDGE('',*,*,#10367,.F.);
#15152=ORIENTED_EDGE('',*,*,#10395,.F.);
#15153=ORIENTED_EDGE('',*,*,#10302,.F.);
#15154=ORIENTED_EDGE('',*,*,#10392,.T.);
#15155=ORIENTED_EDGE('',*,*,#10303,.F.);
#15156=ORIENTED_EDGE('',*,*,#10396,.F.);
#15157=ORIENTED_EDGE('',*,*,#10338,.F.);
#15158=ORIENTED_EDGE('',*,*,#10393,.T.);
#15159=ORIENTED_EDGE('',*,*,#10349,.F.);
#15160=ORIENTED_EDGE('',*,*,#10397,.F.);
#15161=ORIENTED_EDGE('',*,*,#10324,.F.);
#15162=ORIENTED_EDGE('',*,*,#10394,.T.);
#15163=ORIENTED_EDGE('',*,*,#10326,.F.);
#15164=ORIENTED_EDGE('',*,*,#10398,.F.);
#15165=ORIENTED_EDGE('',*,*,#10357,.F.);
#15166=ORIENTED_EDGE('',*,*,#10395,.T.);
#15167=ORIENTED_EDGE('',*,*,#10366,.F.);
#15168=ORIENTED_EDGE('',*,*,#10399,.F.);
#15169=ORIENTED_EDGE('',*,*,#10298,.F.);
#15170=ORIENTED_EDGE('',*,*,#10400,.F.);
#15171=ORIENTED_EDGE('',*,*,#10299,.F.);
#15172=ORIENTED_EDGE('',*,*,#10401,.F.);
#15173=ORIENTED_EDGE('',*,*,#10293,.F.);
#15174=ORIENTED_EDGE('',*,*,#10396,.T.);
#15175=ORIENTED_EDGE('',*,*,#10300,.F.);
#15176=ORIENTED_EDGE('',*,*,#10402,.F.);
#15177=ORIENTED_EDGE('',*,*,#10339,.F.);
#15178=ORIENTED_EDGE('',*,*,#10397,.T.);
#15179=ORIENTED_EDGE('',*,*,#10348,.F.);
#15180=ORIENTED_EDGE('',*,*,#10403,.F.);
#15181=ORIENTED_EDGE('',*,*,#10327,.F.);
#15182=ORIENTED_EDGE('',*,*,#10398,.T.);
#15183=ORIENTED_EDGE('',*,*,#10329,.F.);
#15184=ORIENTED_EDGE('',*,*,#10404,.F.);
#15185=ORIENTED_EDGE('',*,*,#10358,.F.);
#15186=ORIENTED_EDGE('',*,*,#10401,.T.);
#15187=ORIENTED_EDGE('',*,*,#10399,.T.);
#15188=ORIENTED_EDGE('',*,*,#10405,.F.);
#15189=ORIENTED_EDGE('',*,*,#10402,.T.);
#15190=ORIENTED_EDGE('',*,*,#10400,.T.);
#15191=ORIENTED_EDGE('',*,*,#10406,.F.);
#15192=ORIENTED_EDGE('',*,*,#10403,.T.);
#15193=ORIENTED_EDGE('',*,*,#10347,.F.);
#15194=ORIENTED_EDGE('',*,*,#10407,.F.);
#15195=ORIENTED_EDGE('',*,*,#10330,.F.);
#15196=ORIENTED_EDGE('',*,*,#10404,.T.);
#15197=ORIENTED_EDGE('',*,*,#10332,.F.);
#15198=ORIENTED_EDGE('',*,*,#10408,.F.);
#15199=ORIENTED_EDGE('',*,*,#10359,.F.);
#15200=ORIENTED_EDGE('',*,*,#10405,.T.);
#15201=ORIENTED_EDGE('',*,*,#10365,.F.);
#15202=ORIENTED_EDGE('',*,*,#10409,.F.);
#15203=ORIENTED_EDGE('',*,*,#10294,.F.);
#15204=ORIENTED_EDGE('',*,*,#10410,.F.);
#15205=ORIENTED_EDGE('',*,*,#10295,.F.);
#15206=ORIENTED_EDGE('',*,*,#10411,.F.);
#15207=ORIENTED_EDGE('',*,*,#10289,.F.);
#15208=ORIENTED_EDGE('',*,*,#10406,.T.);
#15209=ORIENTED_EDGE('',*,*,#10296,.F.);
#15210=ORIENTED_EDGE('',*,*,#10412,.F.);
#15211=ORIENTED_EDGE('',*,*,#10340,.F.);
#15212=ORIENTED_EDGE('',*,*,#10407,.T.);
#15213=ORIENTED_EDGE('',*,*,#10346,.F.);
#15214=ORIENTED_EDGE('',*,*,#10413,.F.);
#15215=ORIENTED_EDGE('',*,*,#10333,.F.);
#15216=ORIENTED_EDGE('',*,*,#10414,.F.);
#15217=ORIENTED_EDGE('',*,*,#10331,.F.);
#15218=ORIENTED_EDGE('',*,*,#10415,.F.);
#15219=ORIENTED_EDGE('',*,*,#10336,.F.);
#15220=ORIENTED_EDGE('',*,*,#10408,.T.);
#15221=ORIENTED_EDGE('',*,*,#10414,.T.);
#15222=ORIENTED_EDGE('',*,*,#10416,.F.);
#15223=ORIENTED_EDGE('',*,*,#10360,.T.);
#15224=ORIENTED_EDGE('',*,*,#10409,.T.);
#15225=ORIENTED_EDGE('',*,*,#10364,.T.);
#15226=ORIENTED_EDGE('',*,*,#10417,.F.);
#15227=ORIENTED_EDGE('',*,*,#10411,.T.);
#15228=ORIENTED_EDGE('',*,*,#10412,.T.);
#15229=ORIENTED_EDGE('',*,*,#10410,.T.);
#15230=ORIENTED_EDGE('',*,*,#10418,.F.);
#15231=ORIENTED_EDGE('',*,*,#10341,.T.);
#15232=ORIENTED_EDGE('',*,*,#10413,.T.);
#15233=ORIENTED_EDGE('',*,*,#10345,.T.);
#15234=ORIENTED_EDGE('',*,*,#10419,.F.);
#15235=ORIENTED_EDGE('',*,*,#10415,.T.);
#15236=ORIENTED_EDGE('',*,*,#10416,.T.);
#15237=ORIENTED_EDGE('',*,*,#10335,.F.);
#15238=ORIENTED_EDGE('',*,*,#10420,.F.);
#15239=ORIENTED_EDGE('',*,*,#10361,.F.);
#15240=ORIENTED_EDGE('',*,*,#10417,.T.);
#15241=ORIENTED_EDGE('',*,*,#10363,.F.);
#15242=ORIENTED_EDGE('',*,*,#10421,.F.);
#15243=ORIENTED_EDGE('',*,*,#10290,.F.);
#15244=ORIENTED_EDGE('',*,*,#10418,.T.);
#15245=ORIENTED_EDGE('',*,*,#10292,.F.);
#15246=ORIENTED_EDGE('',*,*,#10422,.F.);
#15247=ORIENTED_EDGE('',*,*,#10342,.F.);
#15248=ORIENTED_EDGE('',*,*,#10419,.T.);
#15249=ORIENTED_EDGE('',*,*,#10344,.F.);
#15250=ORIENTED_EDGE('',*,*,#10423,.F.);
#15251=ORIENTED_EDGE('',*,*,#10337,.F.);
#15252=ORIENTED_EDGE('',*,*,#10362,.T.);
#15253=ORIENTED_EDGE('',*,*,#10420,.T.);
#15254=ORIENTED_EDGE('',*,*,#10424,.F.);
#15255=ORIENTED_EDGE('',*,*,#10421,.T.);
#15256=ORIENTED_EDGE('',*,*,#10343,.T.);
#15257=ORIENTED_EDGE('',*,*,#10422,.T.);
#15258=ORIENTED_EDGE('',*,*,#10425,.F.);
#15259=ORIENTED_EDGE('',*,*,#10423,.T.);
#15260=ORIENTED_EDGE('',*,*,#10424,.T.);
#15261=ORIENTED_EDGE('',*,*,#10334,.F.);
#15262=ORIENTED_EDGE('',*,*,#10425,.T.);
#15263=ORIENTED_EDGE('',*,*,#10291,.F.);
#15264=ORIENTED_EDGE('',*,*,#10379,.F.);
#15265=ORIENTED_EDGE('',*,*,#10426,.T.);
#15266=ORIENTED_EDGE('',*,*,#10375,.F.);
#15267=ORIENTED_EDGE('',*,*,#10426,.F.);
#15268=ORIENTED_EDGE('',*,*,#10376,.F.);
#15269=ORIENTED_EDGE('',*,*,#10377,.F.);
#15270=ORIENTED_EDGE('',*,*,#10427,.T.);
#15271=ORIENTED_EDGE('',*,*,#10356,.F.);
#15272=ORIENTED_EDGE('',*,*,#10427,.F.);
#16591=PLANE('',#18926);
#16592=PLANE('',#18927);
#16593=PLANE('',#18928);
#16594=PLANE('',#18929);
#16595=PLANE('',#18930);
#16596=PLANE('',#18931);
#16597=PLANE('',#18932);
#16598=PLANE('',#18933);
#16599=PLANE('',#18934);
#16600=PLANE('',#18935);
#16601=PLANE('',#18936);
#16602=PLANE('',#18937);
#16603=PLANE('',#18938);
#16604=PLANE('',#18939);
#16605=PLANE('',#18940);
#16606=PLANE('',#18946);
#17341=ADVANCED_FACE('',(#4225),#3361,.T.);
#17342=ADVANCED_FACE('',(#4226),#16591,.F.);
#17343=ADVANCED_FACE('',(#4227),#16592,.F.);
#17344=ADVANCED_FACE('',(#4228),#16593,.F.);
#17345=ADVANCED_FACE('',(#4229),#16594,.F.);
#17346=ADVANCED_FACE('',(#4230),#16595,.F.);
#17347=ADVANCED_FACE('',(#4231),#16596,.F.);
#17348=ADVANCED_FACE('',(#4232),#16597,.F.);
#17349=ADVANCED_FACE('',(#4233),#16598,.F.);
#17350=ADVANCED_FACE('',(#4234),#16599,.F.);
#17351=ADVANCED_FACE('',(#4235),#16600,.F.);
#17352=ADVANCED_FACE('',(#4236),#16601,.F.);
#17353=ADVANCED_FACE('',(#4237),#16602,.F.);
#17354=ADVANCED_FACE('',(#4238),#16603,.F.);
#17355=ADVANCED_FACE('',(#4239),#16604,.F.);
#17356=ADVANCED_FACE('',(#4240,#3508),#16605,.T.);
#17357=ADVANCED_FACE('',(#4241,#3509),#16606,.T.);
#17358=ADVANCED_FACE('',(#4242),#3362,.F.);
#17359=ADVANCED_FACE('',(#4243),#3363,.T.);
#17360=ADVANCED_FACE('',(#4244),#3364,.T.);
#17361=ADVANCED_FACE('',(#4245),#3365,.T.);
#17362=ADVANCED_FACE('',(#4246),#3366,.T.);
#17363=ADVANCED_FACE('',(#4247),#3367,.T.);
#17364=ADVANCED_FACE('',(#4248),#3368,.T.);
#17365=ADVANCED_FACE('',(#4249),#3369,.T.);
#17366=ADVANCED_FACE('',(#4250),#3370,.T.);
#17367=ADVANCED_FACE('',(#4251),#3371,.T.);
#17368=ADVANCED_FACE('',(#4252),#3372,.T.);
#17369=ADVANCED_FACE('',(#4253),#3373,.T.);
#17370=ADVANCED_FACE('',(#4254),#3374,.T.);
#17371=ADVANCED_FACE('',(#4255),#3375,.T.);
#17372=ADVANCED_FACE('',(#4256),#3376,.T.);
#17373=ADVANCED_FACE('',(#4257),#3377,.T.);
#17374=ADVANCED_FACE('',(#4258),#3378,.T.);
#17375=ADVANCED_FACE('',(#4259),#3379,.T.);
#17376=ADVANCED_FACE('',(#4260),#3380,.T.);
#17377=ADVANCED_FACE('',(#4261),#3381,.T.);
#17378=ADVANCED_FACE('',(#4262),#3382,.T.);
#17379=ADVANCED_FACE('',(#4263),#3383,.T.);
#17380=ADVANCED_FACE('',(#4264),#3384,.T.);
#17381=ADVANCED_FACE('',(#4265),#149,.T.);
#17382=ADVANCED_FACE('',(#4266),#150,.T.);
#17383=ADVANCED_FACE('',(#4267),#3385,.T.);
#17384=ADVANCED_FACE('',(#4268),#3386,.T.);
#17385=ADVANCED_FACE('',(#4269),#3387,.T.);
#17386=ADVANCED_FACE('',(#4270),#3388,.F.);
#17387=ADVANCED_FACE('',(#4271),#3389,.T.);
#17388=ADVANCED_FACE('',(#4272),#3390,.T.);
#17389=ADVANCED_FACE('',(#4273),#3391,.F.);
#17390=ADVANCED_FACE('',(#4274),#248,.T.);
#17391=ADVANCED_FACE('',(#4275),#249,.T.);
#17392=ADVANCED_FACE('',(#4276),#250,.T.);
#17393=ADVANCED_FACE('',(#4277),#251,.T.);
#17394=ADVANCED_FACE('',(#4278),#3392,.T.);
#17395=ADVANCED_FACE('',(#4279),#252,.T.);
#17396=ADVANCED_FACE('',(#4280),#253,.T.);
#17397=ADVANCED_FACE('',(#4281),#3393,.T.);
#17398=ADVANCED_FACE('',(#4282),#254,.T.);
#17399=ADVANCED_FACE('',(#4283),#255,.T.);
#17400=ADVANCED_FACE('',(#4284),#3394,.F.);
#17401=ADVANCED_FACE('',(#4285),#256,.T.);
#17402=ADVANCED_FACE('',(#4286),#257,.T.);
#17672=CLOSED_SHELL('',(#17341,#17342,#17343,#17344,#17345,#17346,#17347,
#17348,#17349,#17350,#17351,#17352,#17353,#17354,#17355,#17356,#17357,#17358,
#17359,#17360,#17361,#17362,#17363,#17364,#17365,#17366,#17367,#17368,#17369,
#17370,#17371,#17372,#17373,#17374,#17375,#17376,#17377,#17378,#17379,#17380,
#17381,#17382,#17383,#17384,#17385,#17386,#17387,#17388,#17389,#17390,#17391,
#17392,#17393,#17394,#17395,#17396,#17397,#17398,#17399,#17400,#17401,#17402));
#18922=AXIS2_PLACEMENT_3D('',#48241,#22135,#22136);
#18923=AXIS2_PLACEMENT_3D('',#48242,#22137,#22138);
#18924=AXIS2_PLACEMENT_3D('',#48247,#22140,#22141);
#18925=AXIS2_PLACEMENT_3D('',#48250,#22143,#22144);
#18926=AXIS2_PLACEMENT_3D('',#48251,#22145,#22146);
#18927=AXIS2_PLACEMENT_3D('',#48260,#22151,#22152);
#18928=AXIS2_PLACEMENT_3D('',#48269,#22157,#22158);
#18929=AXIS2_PLACEMENT_3D('',#48275,#22162,#22163);
#18930=AXIS2_PLACEMENT_3D('',#48281,#22167,#22168);
#18931=AXIS2_PLACEMENT_3D('',#48287,#22172,#22173);
#18932=AXIS2_PLACEMENT_3D('',#48293,#22177,#22178);
#18933=AXIS2_PLACEMENT_3D('',#48299,#22182,#22183);
#18934=AXIS2_PLACEMENT_3D('',#48305,#22187,#22188);
#18935=AXIS2_PLACEMENT_3D('',#48311,#22192,#22193);
#18936=AXIS2_PLACEMENT_3D('',#48317,#22197,#22198);
#18937=AXIS2_PLACEMENT_3D('',#48323,#22202,#22203);
#18938=AXIS2_PLACEMENT_3D('',#48329,#22207,#22208);
#18939=AXIS2_PLACEMENT_3D('',#48335,#22212,#22213);
#18940=AXIS2_PLACEMENT_3D('',#48344,#22218,#22219);
#18941=AXIS2_PLACEMENT_3D('',#48353,#22223,#22224);
#18942=AXIS2_PLACEMENT_3D('',#48355,#22225,#22226);
#18943=AXIS2_PLACEMENT_3D('',#48357,#22227,#22228);
#18944=AXIS2_PLACEMENT_3D('',#48361,#22230,#22231);
#18945=AXIS2_PLACEMENT_3D('',#48382,#22242,#22243);
#18946=AXIS2_PLACEMENT_3D('',#48383,#22244,#22245);
#18947=AXIS2_PLACEMENT_3D('',#48392,#22249,#22250);
#18948=AXIS2_PLACEMENT_3D('',#48396,#22252,#22253);
#18949=AXIS2_PLACEMENT_3D('',#48398,#22254,#22255);
#18950=AXIS2_PLACEMENT_3D('',#48400,#22256,#22257);
#18951=AXIS2_PLACEMENT_3D('',#48421,#22268,#22269);
#18952=AXIS2_PLACEMENT_3D('',#48422,#22270,#22271);
#18953=AXIS2_PLACEMENT_3D('',#48425,#22272,#22273);
#18954=AXIS2_PLACEMENT_3D('',#48426,#22274,#22275);
#18955=AXIS2_PLACEMENT_3D('',#48429,#22277,#22278);
#18956=AXIS2_PLACEMENT_3D('',#48430,#22279,#22280);
#18957=AXIS2_PLACEMENT_3D('',#48431,#22281,#22282);
#18958=AXIS2_PLACEMENT_3D('',#48432,#22283,#22284);
#18959=AXIS2_PLACEMENT_3D('',#48433,#22285,#22286);
#18960=AXIS2_PLACEMENT_3D('',#48434,#22287,#22288);
#18961=AXIS2_PLACEMENT_3D('',#48435,#22289,#22290);
#18962=AXIS2_PLACEMENT_3D('',#48436,#22291,#22292);
#18963=AXIS2_PLACEMENT_3D('',#48437,#22293,#22294);
#18964=AXIS2_PLACEMENT_3D('',#48438,#22295,#22296);
#18965=AXIS2_PLACEMENT_3D('',#48439,#22297,#22298);
#18966=AXIS2_PLACEMENT_3D('',#48440,#22299,#22300);
#18967=AXIS2_PLACEMENT_3D('',#48441,#22301,#22302);
#18968=AXIS2_PLACEMENT_3D('',#48442,#22303,#22304);
#18969=AXIS2_PLACEMENT_3D('',#48443,#22305,#22306);
#18970=AXIS2_PLACEMENT_3D('',#48444,#22307,#22308);
#18971=AXIS2_PLACEMENT_3D('',#48445,#22309,#22310);
#18972=AXIS2_PLACEMENT_3D('',#48446,#22311,#22312);
#18973=AXIS2_PLACEMENT_3D('',#48447,#22313,#22314);
#18974=AXIS2_PLACEMENT_3D('',#48448,#22315,#22316);
#18975=AXIS2_PLACEMENT_3D('',#48449,#22317,#22318);
#18976=AXIS2_PLACEMENT_3D('',#48450,#22319,#22320);
#18977=AXIS2_PLACEMENT_3D('',#48451,#22321,#22322);
#18978=AXIS2_PLACEMENT_3D('',#48452,#22323,#22324);
#18979=AXIS2_PLACEMENT_3D('',#48453,#22325,#22326);
#18980=AXIS2_PLACEMENT_3D('',#48454,#22327,#22328);
#18981=AXIS2_PLACEMENT_3D('',#48455,#22329,#22330);
#18982=AXIS2_PLACEMENT_3D('',#48456,#22331,#22332);
#18983=AXIS2_PLACEMENT_3D('',#48457,#22333,#22334);
#18984=AXIS2_PLACEMENT_3D('',#48458,#22335,#22336);
#18985=AXIS2_PLACEMENT_3D('',#48459,#22337,#22338);
#18986=AXIS2_PLACEMENT_3D('',#48460,#22339,#22340);
#18987=AXIS2_PLACEMENT_3D('',#48461,#22341,#22342);
#18988=AXIS2_PLACEMENT_3D('',#48462,#22343,#22344);
#18989=AXIS2_PLACEMENT_3D('',#48463,#22345,#22346);
#18990=AXIS2_PLACEMENT_3D('',#48464,#22347,#22348);
#18991=AXIS2_PLACEMENT_3D('',#48465,#22349,#22350);
#18992=AXIS2_PLACEMENT_3D('',#48466,#22351,#22352);
#18993=AXIS2_PLACEMENT_3D('',#48467,#22353,#22354);
#18994=AXIS2_PLACEMENT_3D('',#48468,#22355,#22356);
#18995=AXIS2_PLACEMENT_3D('',#48469,#22357,#22358);
#18996=AXIS2_PLACEMENT_3D('',#48470,#22359,#22360);
#18997=AXIS2_PLACEMENT_3D('',#48471,#22361,#22362);
#18998=AXIS2_PLACEMENT_3D('',#48472,#22363,#22364);
#18999=AXIS2_PLACEMENT_3D('',#48473,#22365,#22366);
#19000=AXIS2_PLACEMENT_3D('',#48474,#22367,#22368);
#19001=AXIS2_PLACEMENT_3D('',#48475,#22369,#22370);
#19002=AXIS2_PLACEMENT_3D('',#48476,#22371,#22372);
#19003=AXIS2_PLACEMENT_3D('',#48477,#22373,#22374);
#19004=AXIS2_PLACEMENT_3D('',#48478,#22375,#22376);
#19005=AXIS2_PLACEMENT_3D('',#48479,#22377,#22378);
#19006=AXIS2_PLACEMENT_3D('',#48480,#22379,#22380);
#19007=AXIS2_PLACEMENT_3D('',#48481,#22381,#22382);
#19008=AXIS2_PLACEMENT_3D('',#48482,#22383,#22384);
#19009=AXIS2_PLACEMENT_3D('',#48483,#22385,#22386);
#19010=AXIS2_PLACEMENT_3D('',#48484,#22387,#22388);
#19011=AXIS2_PLACEMENT_3D('',#48485,#22389,#22390);
#19012=AXIS2_PLACEMENT_3D('',#48486,#22391,#22392);
#19013=AXIS2_PLACEMENT_3D('',#48487,#22393,#22394);
#19014=AXIS2_PLACEMENT_3D('',#48488,#22395,#22396);
#19015=AXIS2_PLACEMENT_3D('',#48489,#22397,#22398);
#19016=AXIS2_PLACEMENT_3D('',#48490,#22399,#22400);
#19017=AXIS2_PLACEMENT_3D('',#48491,#22401,#22402);
#19018=AXIS2_PLACEMENT_3D('',#48492,#22403,#22404);
#19019=AXIS2_PLACEMENT_3D('',#48493,#22405,#22406);
#19020=AXIS2_PLACEMENT_3D('',#48494,#22407,#22408);
#19021=AXIS2_PLACEMENT_3D('',#48495,#22409,#22410);
#19022=AXIS2_PLACEMENT_3D('',#48496,#22411,#22412);
#19023=AXIS2_PLACEMENT_3D('',#48497,#22413,#22414);
#19024=AXIS2_PLACEMENT_3D('',#48498,#22415,#22416);
#19025=AXIS2_PLACEMENT_3D('',#48499,#22417,#22418);
#19026=AXIS2_PLACEMENT_3D('',#48500,#22419,#22420);
#19027=AXIS2_PLACEMENT_3D('',#48501,#22421,#22422);
#19028=AXIS2_PLACEMENT_3D('',#48502,#22423,#22424);
#19029=AXIS2_PLACEMENT_3D('',#48503,#22425,#22426);
#19030=AXIS2_PLACEMENT_3D('',#48504,#22427,#22428);
#19031=AXIS2_PLACEMENT_3D('',#48505,#22429,#22430);
#19032=AXIS2_PLACEMENT_3D('',#48506,#22431,#22432);
#19033=AXIS2_PLACEMENT_3D('',#48507,#22433,#22434);
#19034=AXIS2_PLACEMENT_3D('',#48508,#22435,#22436);
#19035=AXIS2_PLACEMENT_3D('',#48509,#22437,#22438);
#19036=AXIS2_PLACEMENT_3D('',#48510,#22439,#22440);
#19037=AXIS2_PLACEMENT_3D('',#48511,#22441,#22442);
#19038=AXIS2_PLACEMENT_3D('',#48512,#22443,#22444);
#19039=AXIS2_PLACEMENT_3D('',#48513,#22445,#22446);
#19040=AXIS2_PLACEMENT_3D('',#48514,#22447,#22448);
#19041=AXIS2_PLACEMENT_3D('',#48515,#22449,#22450);
#19042=AXIS2_PLACEMENT_3D('',#48516,#22451,#22452);
#19043=AXIS2_PLACEMENT_3D('',#48517,#22453,#22454);
#19044=AXIS2_PLACEMENT_3D('',#48518,#22455,#22456);
#19045=AXIS2_PLACEMENT_3D('',#48519,#22457,#22458);
#19046=AXIS2_PLACEMENT_3D('',#48520,#22459,#22460);
#19047=AXIS2_PLACEMENT_3D('',#48521,#22461,#22462);
#22135=DIRECTION('axis',(0.,0.,1.));
#22136=DIRECTION('refdir',(1.,0.,0.));
#22137=DIRECTION('center_axis',(0.,1.,0.));
#22138=DIRECTION('ref_axis',(-0.96822474174621,0.,-0.250081685595898));
#22139=DIRECTION('',(0.,1.,0.));
#22140=DIRECTION('center_axis',(0.,-1.,0.));
#22141=DIRECTION('ref_axis',(0.,0.,-1.));
#22142=DIRECTION('',(0.,1.,0.));
#22143=DIRECTION('center_axis',(0.,1.,0.));
#22144=DIRECTION('ref_axis',(0.,0.,1.));
#22145=DIRECTION('center_axis',(0.432457515077943,0.,0.901654311614274));
#22146=DIRECTION('ref_axis',(0.901654311614274,0.,-0.432457515077943));
#22147=DIRECTION('',(0.,1.,0.));
#22148=DIRECTION('',(0.901654311614274,0.,-0.432457515077943));
#22149=DIRECTION('',(0.,-1.,0.));
#22150=DIRECTION('',(0.901654311614274,0.,-0.432457515077943));
#22151=DIRECTION('center_axis',(0.296407207072259,0.,0.955061656436705));
#22152=DIRECTION('ref_axis',(0.955061656436705,0.,-0.296407207072259));
#22153=DIRECTION('',(0.,1.,0.));
#22154=DIRECTION('',(0.955061656436705,0.,-0.296407207072259));
#22155=DIRECTION('',(0.,1.,0.));
#22156=DIRECTION('',(0.955061656436705,0.,-0.296407207072259));
#22157=DIRECTION('center_axis',(-0.931114934364932,0.,0.364725895711544));
#22158=DIRECTION('ref_axis',(0.364725895711544,0.,0.931114934364932));
#22159=DIRECTION('',(0.,1.,0.));
#22160=DIRECTION('',(0.364725895711544,0.,0.931114934364932));
#22161=DIRECTION('',(0.364725895711544,0.,0.931114934364932));
#22162=DIRECTION('center_axis',(-0.735023390931532,0.,-0.678041750029829));
#22163=DIRECTION('ref_axis',(-0.678041750029829,0.,0.735023390931532));
#22164=DIRECTION('',(0.,1.,0.));
#22165=DIRECTION('',(-0.678041750029829,0.,0.735023390931532));
#22166=DIRECTION('',(-0.678041750029829,0.,0.735023390931532));
#22167=DIRECTION('center_axis',(0.288569434854979,0.,-0.957458971062195));
#22168=DIRECTION('ref_axis',(-0.957458971062195,0.,-0.288569434854979));
#22169=DIRECTION('',(0.,1.,0.));
#22170=DIRECTION('',(-0.957458971062196,0.,-0.288569434854979));
#22171=DIRECTION('',(-0.957458971062196,0.,-0.288569434854979));
#22172=DIRECTION('center_axis',(-0.779581087140967,0.,-0.626301308135395));
#22173=DIRECTION('ref_axis',(-0.626301308135395,0.,0.779581087140967));
#22174=DIRECTION('',(0.,1.,0.));
#22175=DIRECTION('',(-0.626301308135395,0.,0.779581087140967));
#22176=DIRECTION('',(-0.626301308135395,0.,0.779581087140967));
#22177=DIRECTION('center_axis',(-0.872778976562211,0.,0.488115619572884));
#22178=DIRECTION('ref_axis',(0.488115619572884,0.,0.872778976562211));
#22179=DIRECTION('',(0.,1.,0.));
#22180=DIRECTION('',(0.488115619572884,0.,0.872778976562211));
#22181=DIRECTION('',(0.488115619572884,0.,0.872778976562211));
#22182=DIRECTION('center_axis',(-0.82050401645276,0.,-0.571640760429912));
#22183=DIRECTION('ref_axis',(-0.571640760429912,0.,0.82050401645276));
#22184=DIRECTION('',(0.,1.,0.));
#22185=DIRECTION('',(-0.571640760429912,0.,0.82050401645276));
#22186=DIRECTION('',(-0.571640760429912,0.,0.82050401645276));
#22187=DIRECTION('center_axis',(0.155507703829795,0.,-0.987834679513523));
#22188=DIRECTION('ref_axis',(-0.987834679513523,0.,-0.155507703829795));
#22189=DIRECTION('',(0.,1.,0.));
#22190=DIRECTION('',(-0.987834679513523,0.,-0.155507703829795));
#22191=DIRECTION('',(-0.987834679513523,0.,-0.155507703829795));
#22192=DIRECTION('center_axis',(-0.857601377279671,0.,-0.514314959619115));
#22193=DIRECTION('ref_axis',(-0.514314959619115,0.,0.857601377279671));
#22194=DIRECTION('',(0.,1.,0.));
#22195=DIRECTION('',(-0.514314959619115,0.,0.857601377279671));
#22196=DIRECTION('',(-0.514314959619115,0.,0.857601377279671));
#22197=DIRECTION('center_axis',(-0.798184797787376,0.,0.6024126729918));
#22198=DIRECTION('ref_axis',(0.6024126729918,0.,0.798184797787376));
#22199=DIRECTION('',(0.,1.,0.));
#22200=DIRECTION('',(0.6024126729918,0.,0.798184797787376));
#22201=DIRECTION('',(0.6024126729918,0.,0.798184797787376));
#22202=DIRECTION('center_axis',(-0.890700204600685,0.,-0.454591185049047));
#22203=DIRECTION('ref_axis',(-0.454591185049047,0.,0.890700204600686));
#22204=DIRECTION('',(0.,1.,0.));
#22205=DIRECTION('',(-0.454591185049047,0.,0.890700204600686));
#22206=DIRECTION('',(-0.454591185049047,0.,0.890700204600686));
#22207=DIRECTION('center_axis',(0.0195491585141347,0.,-0.999808896940505));
#22208=DIRECTION('ref_axis',(-0.999808896940505,0.,-0.0195491585141347));
#22209=DIRECTION('',(0.,1.,0.));
#22210=DIRECTION('',(-0.999808896940505,0.,-0.0195491585141347));
#22211=DIRECTION('',(-0.999808896940505,0.,-0.0195491585141347));
#22212=DIRECTION('center_axis',(-0.305368030084627,0.,-0.952234407172013));
#22213=DIRECTION('ref_axis',(-0.952234407172013,0.,0.305368030084627));
#22214=DIRECTION('',(0.,-1.,0.));
#22215=DIRECTION('',(-0.952234407172013,0.,0.305368030084627));
#22216=DIRECTION('',(0.,1.,0.));
#22217=DIRECTION('',(-0.952234407172013,0.,0.305368030084627));
#22218=DIRECTION('center_axis',(0.,1.,0.));
#22219=DIRECTION('ref_axis',(0.,0.,1.));
#22220=DIRECTION('',(0.364725895711544,0.,0.931114934364932));
#22221=DIRECTION('',(0.955061656436705,0.,-0.296407207072259));
#22222=DIRECTION('',(0.901654311614274,0.,-0.432457515077943));
#22223=DIRECTION('center_axis',(0.,1.,0.));
#22224=DIRECTION('ref_axis',(0.,0.,1.));
#22225=DIRECTION('center_axis',(0.,1.,0.));
#22226=DIRECTION('ref_axis',(0.,0.,1.));
#22227=DIRECTION('center_axis',(0.,1.,0.));
#22228=DIRECTION('ref_axis',(0.,0.,1.));
#22229=DIRECTION('',(-0.952234407172013,0.,0.305368030084627));
#22230=DIRECTION('center_axis',(0.,1.,0.));
#22231=DIRECTION('ref_axis',(0.,0.,1.));
#22232=DIRECTION('',(-0.999808896940505,0.,-0.0195491585141347));
#22233=DIRECTION('',(-0.454591185049047,0.,0.890700204600686));
#22234=DIRECTION('',(0.6024126729918,0.,0.798184797787376));
#22235=DIRECTION('',(-0.514314959619115,0.,0.857601377279671));
#22236=DIRECTION('',(-0.987834679513523,0.,-0.155507703829795));
#22237=DIRECTION('',(-0.571640760429912,0.,0.82050401645276));
#22238=DIRECTION('',(0.488115619572884,0.,0.872778976562211));
#22239=DIRECTION('',(-0.626301308135395,0.,0.779581087140967));
#22240=DIRECTION('',(-0.957458971062196,0.,-0.288569434854979));
#22241=DIRECTION('',(-0.678041750029829,0.,0.735023390931532));
#22242=DIRECTION('center_axis',(0.,1.,0.));
#22243=DIRECTION('ref_axis',(0.,0.,1.));
#22244=DIRECTION('center_axis',(0.,-1.,0.));
#22245=DIRECTION('ref_axis',(0.,0.,-1.));
#22246=DIRECTION('',(0.6024126729918,0.,0.798184797787376));
#22247=DIRECTION('',(-0.454591185049047,0.,0.890700204600686));
#22248=DIRECTION('',(-0.999808896940505,0.,-0.0195491585141347));
#22249=DIRECTION('center_axis',(0.,-1.,0.));
#22250=DIRECTION('ref_axis',(0.,0.,-1.));
#22251=DIRECTION('',(-0.952234407172013,0.,0.305368030084627));
#22252=DIRECTION('center_axis',(0.,-1.,0.));
#22253=DIRECTION('ref_axis',(0.,0.,-1.));
#22254=DIRECTION('center_axis',(0.,-1.,0.));
#22255=DIRECTION('ref_axis',(0.,0.,-1.));
#22256=DIRECTION('center_axis',(0.,-1.,0.));
#22257=DIRECTION('ref_axis',(0.,0.,-1.));
#22258=DIRECTION('',(0.901654311614274,0.,-0.432457515077943));
#22259=DIRECTION('',(0.955061656436705,0.,-0.296407207072259));
#22260=DIRECTION('',(0.364725895711544,0.,0.931114934364932));
#22261=DIRECTION('',(-0.678041750029829,0.,0.735023390931532));
#22262=DIRECTION('',(-0.957458971062196,0.,-0.288569434854979));
#22263=DIRECTION('',(-0.626301308135395,0.,0.779581087140967));
#22264=DIRECTION('',(0.488115619572884,0.,0.872778976562211));
#22265=DIRECTION('',(-0.571640760429912,0.,0.82050401645276));
#22266=DIRECTION('',(-0.987834679513523,0.,-0.155507703829795));
#22267=DIRECTION('',(-0.514314959619115,0.,0.857601377279671));
#22268=DIRECTION('center_axis',(0.,-1.,0.));
#22269=DIRECTION('ref_axis',(0.,0.,-1.));
#22270=DIRECTION('center_axis',(0.,-1.,0.));
#22271=DIRECTION('ref_axis',(0.,0.,-1.));
#22272=DIRECTION('center_axis',(0.,1.,0.));
#22273=DIRECTION('ref_axis',(0.,0.,1.));
#22274=DIRECTION('center_axis',(0.,1.,0.));
#22275=DIRECTION('ref_axis',(0.,0.,1.));
#22276=DIRECTION('',(0.,-1.,0.));
#22277=DIRECTION('center_axis',(0.,-1.,0.));
#22278=DIRECTION('ref_axis',(0.,0.,-1.));
#22279=DIRECTION('center_axis',(-0.488115619572884,0.,-0.872778976562211));
#22280=DIRECTION('ref_axis',(-0.872778976562211,0.,0.488115619572884));
#22281=DIRECTION('center_axis',(0.0492674350094236,0.,-0.998785622567522));
#22282=DIRECTION('ref_axis',(-0.998785622567522,0.,-0.0492674350094236));
#22283=DIRECTION('center_axis',(0.0833383631889745,0.,-0.996521307961341));
#22284=DIRECTION('ref_axis',(-0.996521307961341,0.,-0.0833383631889746));
#22285=DIRECTION('center_axis',(0.626301308135395,0.,-0.779581087140967));
#22286=DIRECTION('ref_axis',(-0.779581087140968,0.,-0.626301308135395));
#22287=DIRECTION('center_axis',(0.955149485630946,0.,-0.29612406200601));
#22288=DIRECTION('ref_axis',(-0.29612406200601,0.,-0.955149485630946));
#22289=DIRECTION('center_axis',(0.626301308135395,0.,-0.779581087140967));
#22290=DIRECTION('ref_axis',(-0.779581087140968,0.,-0.626301308135395));
#22291=DIRECTION('center_axis',(0.955149485630946,0.,-0.29612406200601));
#22292=DIRECTION('ref_axis',(0.29612406200601,0.,0.955149485630946));
#22293=DIRECTION('center_axis',(0.0833383631889745,0.,-0.996521307961341));
#22294=DIRECTION('ref_axis',(0.996521307961341,0.,0.0833383631889746));
#22295=DIRECTION('center_axis',(-0.488115619572884,0.,-0.872778976562211));
#22296=DIRECTION('ref_axis',(-0.872778976562211,0.,0.488115619572884));
#22297=DIRECTION('center_axis',(0.0492674350094236,0.,-0.998785622567522));
#22298=DIRECTION('ref_axis',(0.998785622567522,0.,0.0492674350094236));
#22299=DIRECTION('center_axis',(0.571640760429912,0.,-0.82050401645276));
#22300=DIRECTION('ref_axis',(-0.82050401645276,0.,-0.571640760429912));
#22301=DIRECTION('center_axis',(0.919859028046646,0.,-0.392249115385974));
#22302=DIRECTION('ref_axis',(-0.392249115385974,0.,-0.919859028046646));
#22303=DIRECTION('center_axis',(0.957458971062196,0.,0.288569434854979));
#22304=DIRECTION('ref_axis',(0.288569434854979,0.,-0.957458971062195));
#22305=DIRECTION('center_axis',(0.964702659073528,0.,-0.263341564468019));
#22306=DIRECTION('ref_axis',(-0.263341564468019,0.,-0.964702659073528));
#22307=DIRECTION('center_axis',(0.957458971062196,0.,0.288569434854979));
#22308=DIRECTION('ref_axis',(0.288569434854979,0.,-0.957458971062195));
#22309=DIRECTION('center_axis',(0.964702659073528,0.,-0.263341564468019));
#22310=DIRECTION('ref_axis',(0.263341564468019,0.,0.964702659073528));
#22311=DIRECTION('center_axis',(0.571640760429912,0.,-0.82050401645276));
#22312=DIRECTION('ref_axis',(-0.82050401645276,0.,-0.571640760429912));
#22313=DIRECTION('center_axis',(0.919859028046646,0.,-0.392249115385974));
#22314=DIRECTION('ref_axis',(0.392249115385974,0.,0.919859028046646));
#22315=DIRECTION('center_axis',(0.987834679513523,0.,0.155507703829795));
#22316=DIRECTION('ref_axis',(0.155507703829795,0.,-0.987834679513523));
#22317=DIRECTION('center_axis',(0.905930950538282,0.,-0.423425451356913));
#22318=DIRECTION('ref_axis',(-0.423425451356913,0.,-0.905930950538282));
#22319=DIRECTION('center_axis',(0.678041750029829,0.,-0.735023390931532));
#22320=DIRECTION('ref_axis',(-0.735023390931532,0.,-0.678041750029829));
#22321=DIRECTION('center_axis',(0.184809846851629,0.,-0.982774297845989));
#22322=DIRECTION('ref_axis',(-0.982774297845989,0.,-0.184809846851629));
#22323=DIRECTION('center_axis',(0.678041750029829,0.,-0.735023390931532));
#22324=DIRECTION('ref_axis',(-0.735023390931532,0.,-0.678041750029829));
#22325=DIRECTION('center_axis',(0.184809846851629,0.,-0.982774297845989));
#22326=DIRECTION('ref_axis',(0.982774297845989,0.,0.184809846851629));
#22327=DIRECTION('center_axis',(0.987834679513523,0.,0.155507703829795));
#22328=DIRECTION('ref_axis',(0.155507703829795,0.,-0.987834679513523));
#22329=DIRECTION('center_axis',(0.905930950538282,0.,-0.423425451356913));
#22330=DIRECTION('ref_axis',(0.423425451356913,0.,0.905930950538282));
#22331=DIRECTION('center_axis',(0.514314959619115,0.,-0.857601377279671));
#22332=DIRECTION('ref_axis',(-0.857601377279671,0.,-0.514314959619115));
#22333=DIRECTION('center_axis',(-0.0531308220811139,0.,-0.998587560379652));
#22334=DIRECTION('ref_axis',(-0.998587560379652,0.,0.0531308220811139));
#22335=DIRECTION('center_axis',(-0.364725895711544,0.,-0.931114934364932));
#22336=DIRECTION('ref_axis',(-0.931114934364932,0.,0.364725895711544));
#22337=DIRECTION('center_axis',(-0.90120055904943,0.,-0.433402298527587));
#22338=DIRECTION('ref_axis',(-0.433402298527587,0.,0.90120055904943));
#22339=DIRECTION('center_axis',(-0.364725895711544,0.,-0.931114934364932));
#22340=DIRECTION('ref_axis',(-0.931114934364932,0.,0.364725895711544));
#22341=DIRECTION('center_axis',(-0.90120055904943,0.,-0.433402298527587));
#22342=DIRECTION('ref_axis',(0.433402298527587,0.,-0.90120055904943));
#22343=DIRECTION('center_axis',(0.514314959619115,0.,-0.857601377279671));
#22344=DIRECTION('ref_axis',(-0.857601377279671,0.,-0.514314959619115));
#22345=DIRECTION('center_axis',(-0.0531308220811139,0.,-0.998587560379652));
#22346=DIRECTION('ref_axis',(0.998587560379652,0.,-0.0531308220811139));
#22347=DIRECTION('center_axis',(-0.6024126729918,0.,-0.798184797787376));
#22348=DIRECTION('ref_axis',(-0.798184797787376,0.,0.6024126729918));
#22349=DIRECTION('center_axis',(-0.087192735929436,0.,-0.996191460915591));
#22350=DIRECTION('ref_axis',(-0.996191460915591,0.,0.087192735929436));
#22351=DIRECTION('center_axis',(-0.955061656436705,0.,0.296407207072259));
#22352=DIRECTION('ref_axis',(0.296407207072259,0.,0.955061656436705));
#22353=DIRECTION('center_axis',(-0.955061656436705,2.56262108120603E-13,
0.29640720707226));
#22354=DIRECTION('ref_axis',(0.29640720707226,-1.35902423770987E-29,0.955061656436705));
#22355=DIRECTION('center_axis',(0.,1.,0.));
#22356=DIRECTION('ref_axis',(0.,0.,1.));
#22357=DIRECTION('center_axis',(0.,1.,0.));
#22358=DIRECTION('ref_axis',(0.,0.,1.));
#22359=DIRECTION('center_axis',(0.,-1.,0.));
#22360=DIRECTION('ref_axis',(0.,0.,-1.));
#22361=DIRECTION('center_axis',(-0.955061656436705,0.,0.296407207072259));
#22362=DIRECTION('ref_axis',(0.296407207072259,0.,0.955061656436705));
#22363=DIRECTION('center_axis',(-0.955061656436693,0.,0.296407207072297));
#22364=DIRECTION('ref_axis',(0.296407207072297,0.,0.955061656436693));
#22365=DIRECTION('center_axis',(-0.6024126729918,0.,-0.798184797787376));
#22366=DIRECTION('ref_axis',(-0.798184797787376,0.,0.6024126729918));
#22367=DIRECTION('center_axis',(-0.087192735929436,0.,-0.996191460915591));
#22368=DIRECTION('ref_axis',(0.996191460915591,0.,-0.087192735929436));
#22369=DIRECTION('center_axis',(0.454591185049047,0.,-0.890700204600686));
#22370=DIRECTION('ref_axis',(-0.890700204600686,0.,-0.454591185049047));
#22371=DIRECTION('center_axis',(0.857880163767375,0.,-0.513849807448113));
#22372=DIRECTION('ref_axis',(-0.513849807448113,0.,-0.857880163767375));
#22373=DIRECTION('center_axis',(-2.49773075486348E-13,-1.,1.04083408558608E-13));
#22374=DIRECTION('ref_axis',(1.,-2.49366499671666E-13,0.));
#22375=DIRECTION('center_axis',(0.901654311614385,0.,-0.432457515077713));
#22376=DIRECTION('ref_axis',(-0.432457515077713,0.,-0.901654311614385));
#22377=DIRECTION('center_axis',(3.92345661168194E-14,1.,-1.73472347597682E-14));
#22378=DIRECTION('ref_axis',(-1.,3.46944695195361E-14,0.));
#22379=DIRECTION('center_axis',(0.901654311614274,-3.98841325780622E-14,
-0.432457515077943));
#22380=DIRECTION('ref_axis',(-0.432457515077943,1.86255736537329E-29,-0.901654311614274));
#22381=DIRECTION('center_axis',(0.454591185049047,0.,-0.890700204600686));
#22382=DIRECTION('ref_axis',(-0.890700204600686,0.,-0.454591185049047));
#22383=DIRECTION('center_axis',(0.857880163767375,0.,-0.513849807448113));
#22384=DIRECTION('ref_axis',(0.513849807448113,0.,0.857880163767375));
#22385=DIRECTION('center_axis',(0.999808896940505,0.,0.0195491585141347));
#22386=DIRECTION('ref_axis',(0.0195491585141347,0.,-0.999808896940505));
#22387=DIRECTION('center_axis',(-0.999808896940505,0.,-0.0195491585141356));
#22388=DIRECTION('ref_axis',(-0.0195491585141356,0.,0.999808896940505));
#22389=DIRECTION('center_axis',(-0.901654311614274,0.,0.432457515077943));
#22390=DIRECTION('ref_axis',(0.432457515077943,0.,0.901654311614274));
#22391=DIRECTION('center_axis',(-0.901654311614274,3.18662470181932E-16,
0.432457515077943));
#22392=DIRECTION('ref_axis',(0.432457515077943,9.83362535564581E-33,0.901654311614274));
#22393=DIRECTION('center_axis',(0.,1.,0.));
#22394=DIRECTION('ref_axis',(0.,0.,1.));
#22395=DIRECTION('center_axis',(0.,1.,0.));
#22396=DIRECTION('ref_axis',(0.,0.,1.));
#22397=DIRECTION('center_axis',(0.,-1.,0.));
#22398=DIRECTION('ref_axis',(0.,0.,-1.));
#22399=DIRECTION('center_axis',(-0.901654311614274,0.,0.432457515077943));
#22400=DIRECTION('ref_axis',(0.432457515077943,0.,0.901654311614274));
#22401=DIRECTION('center_axis',(-0.901654311614275,0.,0.432457515077941));
#22402=DIRECTION('ref_axis',(0.432457515077941,0.,0.901654311614275));
#22403=DIRECTION('center_axis',(0.999808896940505,0.,0.0195491585141347));
#22404=DIRECTION('ref_axis',(0.0195491585141347,0.,-0.999808896940505));
#22405=DIRECTION('center_axis',(-0.999808896940505,0.,-0.0195491585141356));
#22406=DIRECTION('ref_axis',(-0.0195491585141356,0.,0.999808896940505));
#22407=DIRECTION('center_axis',(0.,-1.,0.));
#22408=DIRECTION('ref_axis',(0.,0.,-1.));
#22409=DIRECTION('center_axis',(0.,-1.,0.));
#22410=DIRECTION('ref_axis',(0.,0.,-1.));
#22411=DIRECTION('center_axis',(0.,1.,0.));
#22412=DIRECTION('ref_axis',(0.,0.,1.));
#22413=DIRECTION('center_axis',(0.,-1.,0.));
#22414=DIRECTION('ref_axis',(0.,0.,-1.));
#22415=DIRECTION('center_axis',(0.952234407172013,1.4810129988824E-15,-0.305368030084626));
#22416=DIRECTION('ref_axis',(-0.305368030084626,-8.45556637047479E-33,-0.952234407172013));
#22417=DIRECTION('center_axis',(0.,-1.,0.));
#22418=DIRECTION('ref_axis',(-0.302115636055689,0.,0.95327128481386));
#22419=DIRECTION('center_axis',(0.48796543950748,0.,0.872862950208262));
#22420=DIRECTION('ref_axis',(0.872862950208263,0.,-0.48796543950748));
#22421=DIRECTION('center_axis',(0.,1.,0.));
#22422=DIRECTION('ref_axis',(0.,0.,1.));
#22423=DIRECTION('center_axis',(0.487965439507477,-3.78543962759172E-15,
0.872862950208264));
#22424=DIRECTION('ref_axis',(0.872862950208264,-1.01742962109045E-31,-0.487965439507477));
#22425=DIRECTION('center_axis',(0.,1.,0.));
#22426=DIRECTION('ref_axis',(-0.144875601312395,0.,-0.989449877530121));
#22427=DIRECTION('center_axis',(0.952234407172013,0.,-0.305368030084625));
#22428=DIRECTION('ref_axis',(-0.305368030084625,0.,-0.952234407172013));
#22429=DIRECTION('center_axis',(0.952234407172013,0.,-0.305368030084627));
#22430=DIRECTION('ref_axis',(-0.305368030084627,0.,-0.952234407172013));
#22431=DIRECTION('center_axis',(-0.952234407172011,0.,0.305368030084631));
#22432=DIRECTION('ref_axis',(0.305368030084631,0.,0.952234407172011));
#22433=DIRECTION('center_axis',(0.,-1.,0.));
#22434=DIRECTION('ref_axis',(-0.96822474174621,0.,-0.250081685595898));
#22435=DIRECTION('center_axis',(0.849631715069657,0.,-0.527376477241631));
#22436=DIRECTION('ref_axis',(-0.527376477241631,0.,-0.849631715069657));
#22437=DIRECTION('center_axis',(0.,1.,0.));
#22438=DIRECTION('ref_axis',(-0.96822474174621,0.,-0.250081685595898));
#22439=DIRECTION('center_axis',(0.849631715069657,0.,-0.527376477241631));
#22440=DIRECTION('ref_axis',(-0.527376477241631,0.,-0.849631715069657));
#22441=DIRECTION('center_axis',(0.952234407172013,0.,-0.305368030084627));
#22442=DIRECTION('ref_axis',(-0.305368030084627,0.,-0.952234407172013));
#22443=DIRECTION('center_axis',(-0.952234407172012,0.,0.30536803008463));
#22444=DIRECTION('ref_axis',(0.30536803008463,0.,0.952234407172012));
#22445=DIRECTION('center_axis',(0.,-1.,0.));
#22446=DIRECTION('ref_axis',(0.,0.,-1.));
#22447=DIRECTION('center_axis',(0.,-1.,0.));
#22448=DIRECTION('ref_axis',(0.,0.,-1.));
#22449=DIRECTION('center_axis',(0.,1.,0.));
#22450=DIRECTION('ref_axis',(0.,0.,1.));
#22451=DIRECTION('center_axis',(0.,1.,0.));
#22452=DIRECTION('ref_axis',(0.,0.,1.));
#22453=DIRECTION('center_axis',(0.,1.,0.));
#22454=DIRECTION('ref_axis',(0.,0.,1.));
#22455=DIRECTION('center_axis',(0.,-1.,0.));
#22456=DIRECTION('ref_axis',(0.,0.,-1.));
#22457=DIRECTION('center_axis',(-1.,0.,0.));
#22458=DIRECTION('ref_axis',(0.,0.,1.));
#22459=DIRECTION('center_axis',(0.,1.,0.));
#22460=DIRECTION('ref_axis',(0.,0.,1.));
#22461=DIRECTION('center_axis',(-1.,0.,0.));
#22462=DIRECTION('ref_axis',(0.,0.,-1.));
#48241=CARTESIAN_POINT('',(0.,0.,0.));
#48242=CARTESIAN_POINT('Origin',(-0.00926982557395217,-0.0158951219150417,
-0.003));
#48243=CARTESIAN_POINT('',(-0.00796053114863977,0.0129,-0.00373194815926121));
#48244=CARTESIAN_POINT('',(-0.00796053114863977,0.0011,-0.00373194815926121));
#48245=CARTESIAN_POINT('',(-0.00796053114863977,-0.0158951219150417,-0.00373194815926121));
#48246=CARTESIAN_POINT('',(-0.00847876085808972,0.0011,-0.00172555242739552));
#48247=CARTESIAN_POINT('Origin',(-0.00926982557395217,0.0011,-0.003));
#48248=CARTESIAN_POINT('',(-0.00847876085808972,0.0129,-0.00172555242739552));
#48249=CARTESIAN_POINT('',(-0.00847876085808972,-0.0158951219150417,-0.00172555242739552));
#48250=CARTESIAN_POINT('Origin',(-0.00926982557395217,0.0129,-0.003));
#48251=CARTESIAN_POINT('Origin',(8.56902727468245E-6,-0.0158951219150417,
-0.00745016612406076));
#48252=CARTESIAN_POINT('',(1.96218223641792E-6,0.0129,-0.00744699730453541));
#48253=CARTESIAN_POINT('',(1.96218223641796E-6,0.0011,-0.00744699730453541));
#48254=CARTESIAN_POINT('',(1.96218223641796E-6,-0.0158951219150417,-0.00744699730453541));
#48255=CARTESIAN_POINT('',(-0.00782999910211115,0.0011,-0.00369057927205054));
#48256=CARTESIAN_POINT('',(-0.00791734410653075,0.0011,-0.00364868627261692));
#48257=CARTESIAN_POINT('',(-0.00782999910211115,0.0129,-0.00369057927205054));
#48258=CARTESIAN_POINT('',(-0.00782999910211115,0.013,-0.00369057927205053));
#48259=CARTESIAN_POINT('',(8.56902727468244E-6,0.0129,-0.00745016612406076));
#48260=CARTESIAN_POINT('Origin',(0.0040613112974471,-0.0158951219150417,
-0.00870795090600599));
#48261=CARTESIAN_POINT('',(0.0040613112974471,0.0011,-0.00870795090600599));
#48262=CARTESIAN_POINT('',(0.0040613112974471,0.0129,-0.00870795090600599));
#48263=CARTESIAN_POINT('',(0.0040613112974471,-0.0158951219150417,-0.00870795090600599));
#48264=CARTESIAN_POINT('',(1.55672130369862E-5,0.0011,-0.00745233803901766));
#48265=CARTESIAN_POINT('',(8.56902727468726E-6,0.0011,-0.00745016612406076));
#48266=CARTESIAN_POINT('',(1.55672130369862E-5,0.0129,-0.00745233803901766));
#48267=CARTESIAN_POINT('',(1.55672130369867E-5,-0.0158951219150417,-0.00745233803901766));
#48268=CARTESIAN_POINT('',(0.0040613112974471,0.0129,-0.00870795090600599));
#48269=CARTESIAN_POINT('Origin',(0.00451057325136412,-0.0158951219150417,
-0.007561022432726));
#48270=CARTESIAN_POINT('',(0.00451057325136412,0.0011,-0.007561022432726));
#48271=CARTESIAN_POINT('',(0.00451057325136412,0.0129,-0.007561022432726));
#48272=CARTESIAN_POINT('',(0.00451057325136412,-0.0158951219150417,-0.007561022432726));
#48273=CARTESIAN_POINT('',(0.0040613112974471,0.0011,-0.00870795090600599));
#48274=CARTESIAN_POINT('',(0.00451057325136412,0.0129,-0.007561022432726));
#48275=CARTESIAN_POINT('Origin',(0.00432022868869639,-0.0158951219150417,
-0.00735468159030551));
#48276=CARTESIAN_POINT('',(0.00432022868869639,0.0011,-0.00735468159030551));
#48277=CARTESIAN_POINT('',(0.00432022868869639,0.0129,-0.00735468159030551));
#48278=CARTESIAN_POINT('',(0.00432022868869639,-0.0158951219150417,-0.00735468159030551));
#48279=CARTESIAN_POINT('',(0.00451057325136413,0.0011,-0.007561022432726));
#48280=CARTESIAN_POINT('',(0.00432022868869639,0.0129,-0.00735468159030551));
#48281=CARTESIAN_POINT('Origin',(0.00314085016583167,-0.0158951219150417,
-0.0077101355618168));
#48282=CARTESIAN_POINT('',(0.00314085016583167,0.0011,-0.0077101355618168));
#48283=CARTESIAN_POINT('',(0.00314085016583167,0.0129,-0.0077101355618168));
#48284=CARTESIAN_POINT('',(0.00314085016583167,-0.0158951219150417,-0.0077101355618168));
#48285=CARTESIAN_POINT('',(0.00432022868869639,0.0011,-0.00735468159030551));
#48286=CARTESIAN_POINT('',(0.00314085016583167,0.0129,-0.0077101355618168));
#48287=CARTESIAN_POINT('Origin',(0.00295417720403981,-0.0158951219150417,
-0.00747777661796151));
#48288=CARTESIAN_POINT('',(0.00295417720403981,0.0011,-0.00747777661796151));
#48289=CARTESIAN_POINT('',(0.00295417720403981,0.0129,-0.00747777661796151));
#48290=CARTESIAN_POINT('',(0.00295417720403981,-0.0158951219150417,-0.00747777661796151));
#48291=CARTESIAN_POINT('',(0.00314085016583167,0.0011,-0.0077101355618168));
#48292=CARTESIAN_POINT('',(0.00295417720403981,0.0129,-0.00747777661796151));
#48293=CARTESIAN_POINT('Origin',(0.00355542811483384,-0.0158951219150417,
-0.00640270519320544));
#48294=CARTESIAN_POINT('',(0.00355542811483384,0.0011,-0.00640270519320544));
#48295=CARTESIAN_POINT('',(0.00355542811483384,0.0129,-0.00640270519320544));
#48296=CARTESIAN_POINT('',(0.00355542811483384,-0.0158951219150417,-0.00640270519320544));
#48297=CARTESIAN_POINT('',(0.00295417720403981,0.0011,-0.00747777661796151));
#48298=CARTESIAN_POINT('',(0.00355542811483384,0.0129,-0.00640270519320544));
#48299=CARTESIAN_POINT('Origin',(0.00339495317277858,-0.0158951219150417,
-0.00617236763925401));
#48300=CARTESIAN_POINT('',(0.00339495317277858,0.0011,-0.00617236763925401));
#48301=CARTESIAN_POINT('',(0.00339495317277858,0.0129,-0.00617236763925401));
#48302=CARTESIAN_POINT('',(0.00339495317277858,-0.0158951219150417,-0.00617236763925401));
#48303=CARTESIAN_POINT('',(0.00355542811483384,0.0011,-0.00640270519320544));
#48304=CARTESIAN_POINT('',(0.00339495317277858,0.0129,-0.00617236763925401));
#48305=CARTESIAN_POINT('Origin',(0.00217815846891078,-0.0158951219150417,
-0.00636391887181847));
#48306=CARTESIAN_POINT('',(0.00217815846891078,0.0011,-0.00636391887181847));
#48307=CARTESIAN_POINT('',(0.00217815846891078,0.0129,-0.00636391887181847));
#48308=CARTESIAN_POINT('',(0.00217815846891078,-0.0158951219150417,-0.00636391887181847));
#48309=CARTESIAN_POINT('',(0.00339495317277858,0.0011,-0.00617236763925401));
#48310=CARTESIAN_POINT('',(0.00217815846891078,0.0129,-0.00636391887181847));
#48311=CARTESIAN_POINT('Origin',(0.00202486372793092,-0.0158951219150417,
-0.00610830550002113));
#48312=CARTESIAN_POINT('',(0.00202486372793092,0.0011,-0.00610830550002113));
#48313=CARTESIAN_POINT('',(0.00202486372793092,0.0129,-0.00610830550002113));
#48314=CARTESIAN_POINT('',(0.00202486372793092,-0.0158951219150417,-0.00610830550002113));
#48315=CARTESIAN_POINT('',(0.00217815846891078,0.0011,-0.00636391887181847));
#48316=CARTESIAN_POINT('',(0.00202486372793092,0.0129,-0.00610830550002113));
#48317=CARTESIAN_POINT('Origin',(0.00276690342874427,-0.0158951219150417,
-0.00512511767031892));
#48318=CARTESIAN_POINT('',(0.00276690342874427,0.0011,-0.00512511767031892));
#48319=CARTESIAN_POINT('',(0.00276690342874427,0.0129,-0.00512511767031892));
#48320=CARTESIAN_POINT('',(0.00276690342874427,-0.0158951219150417,-0.00512511767031892));
#48321=CARTESIAN_POINT('',(0.00202486372793092,0.0011,-0.00610830550002113));
#48322=CARTESIAN_POINT('',(0.00276690342874427,0.0129,-0.00512511767031892));
#48323=CARTESIAN_POINT('Origin',(0.00263928745184173,-0.0158951219150417,
-0.00487507415765127));
#48324=CARTESIAN_POINT('',(0.00263928745184173,0.0011,-0.00487507415765127));
#48325=CARTESIAN_POINT('',(0.00263928745184173,0.0129,-0.00487507415765127));
#48326=CARTESIAN_POINT('',(0.00263928745184173,-0.0158951219150417,-0.00487507415765127));
#48327=CARTESIAN_POINT('',(0.00276690342874427,0.0011,-0.00512511767031893));
#48328=CARTESIAN_POINT('',(0.00263928745184173,0.0129,-0.00487507415765127));
#48329=CARTESIAN_POINT('Origin',(0.0014077431500399,-0.0158951219150417,
-0.00489915441423508));
#48330=CARTESIAN_POINT('',(0.0014243849476499,0.0129,-0.0048988290189116));
#48331=CARTESIAN_POINT('',(0.0014243849476499,0.0011,-0.0048988290189116));
#48332=CARTESIAN_POINT('',(0.0014243849476499,0.001,-0.0048988290189116));
#48333=CARTESIAN_POINT('',(0.00263928745184173,0.0011,-0.00487507415765127));
#48334=CARTESIAN_POINT('',(0.0014077431500399,0.0129,-0.00489915441423508));
#48335=CARTESIAN_POINT('Origin',(-0.00846848477354713,-0.0158951219150417,
-0.00173198859563243));
#48336=CARTESIAN_POINT('',(-0.00845656001337402,0.0129,-0.00173581269660575));
#48337=CARTESIAN_POINT('',(-0.00845656001337402,0.0011,-0.00173581269660575));
#48338=CARTESIAN_POINT('',(-0.00845656001337402,0.001,-0.00173581269660575));
#48339=CARTESIAN_POINT('',(0.00139189322879002,0.0011,-0.00489407156993475));
#48340=CARTESIAN_POINT('',(0.0014077431500399,0.0011,-0.00489915441423508));
#48341=CARTESIAN_POINT('',(0.00139189322879002,0.0129,-0.00489407156993475));
#48342=CARTESIAN_POINT('',(0.00139189322879002,0.013,-0.00489407156993475));
#48343=CARTESIAN_POINT('',(-0.00846848477354713,0.0129,-0.00173198859563243));
#48344=CARTESIAN_POINT('Origin',(-0.00926982557395217,0.013,-0.003));
#48345=CARTESIAN_POINT('',(0.00439463505993757,0.013,-0.00758282450818601));
#48346=CARTESIAN_POINT('',(0.00400212262074066,0.013,-0.00858487618139458));
#48347=CARTESIAN_POINT('',(0.0039681998040106,0.013,-0.00867147831643483));
#48348=CARTESIAN_POINT('',(4.52079337442158E-5,0.013,-0.00735683187337399));
#48349=CARTESIAN_POINT('',(3.82097479819073E-5,0.013,-0.00735465995841708));
#48350=CARTESIAN_POINT('',(-0.00778675335060335,0.013,-0.00360041384088911));
#48351=CARTESIAN_POINT('',(-0.00787409835502296,0.013,-0.00355852084145549));
#48352=CARTESIAN_POINT('',(-0.00804781744366059,0.013,-0.00368315161531047));
#48353=CARTESIAN_POINT('Origin',(-0.00787324485361894,0.013,-0.00378074470321196));
#48354=CARTESIAN_POINT('',(-0.00853149850581388,0.013,-0.00181051559890248));
#48355=CARTESIAN_POINT('Origin',(-0.00926982557395217,0.013,-0.003));
#48356=CARTESIAN_POINT('',(-0.00848709681638249,0.013,-0.00183103613732295));
#48357=CARTESIAN_POINT('Origin',(-0.00842602321036556,0.013,-0.00164058925588855));
#48358=CARTESIAN_POINT('',(0.00136135642578156,0.013,-0.00498929501065195));
#48359=CARTESIAN_POINT('',(0.00137720634703143,0.013,-0.00499437785495228));
#48360=CARTESIAN_POINT('',(0.00142633986350131,0.013,-0.00499880990860565));
#48361=CARTESIAN_POINT('Origin',(0.00142243003179848,0.013,-0.00479884812921755));
#48362=CARTESIAN_POINT('',(0.00257866842927369,0.013,-0.00497627854900125));
#48363=CARTESIAN_POINT('',(0.00264124236769314,0.013,-0.00497505504734532));
#48364=CARTESIAN_POINT('',(0.00264938241039218,0.013,-0.00511483151597876));
#48365=CARTESIAN_POINT('',(0.0026778334082842,0.013,-0.00517057678882383));
#48366=CARTESIAN_POINT('',(0.00190441615676979,0.013,-0.00610189696988579));
#48367=CARTESIAN_POINT('',(0.00194504524815218,0.013,-0.00604806423272195));
#48368=CARTESIAN_POINT('',(0.00212708576461598,0.013,-0.00647319039387763));
#48369=CARTESIAN_POINT('',(0.00209239833118282,0.013,-0.00641535036778038));
#48370=CARTESIAN_POINT('',(0.00334867942190192,0.013,-0.00628088369661617));
#48371=CARTESIAN_POINT('',(0.00341050394316157,0.013,-0.00627115110720536));
#48372=CARTESIAN_POINT('',(0.00343760106241995,0.013,-0.00640851728792926));
#48373=CARTESIAN_POINT('',(0.00347337771318856,0.013,-0.00645986926924843));
#48374=CARTESIAN_POINT('',(0.00283397885998211,0.013,-0.00748782871937848));
#48375=CARTESIAN_POINT('',(0.00286689930638359,0.013,-0.00742896505600422));
#48376=CARTESIAN_POINT('',(0.00310513229246118,0.013,-0.00782534372202691));
#48377=CARTESIAN_POINT('',(0.00306289205711758,0.013,-0.00777276569263034));
#48378=CARTESIAN_POINT('',(0.00428916220193663,0.013,-0.00746848786485147));
#48379=CARTESIAN_POINT('',(0.00434908563218188,0.013,-0.00745042748741173));
#48380=CARTESIAN_POINT('',(0.00443707091227097,0.013,-0.00762882660772898));
#48381=CARTESIAN_POINT('',(-0.00926982557395217,0.013,-0.0036));
#48382=CARTESIAN_POINT('Origin',(-0.00926982557395217,0.013,-0.003));
#48383=CARTESIAN_POINT('Origin',(-0.00926982557395217,0.001,0.003));
#48384=CARTESIAN_POINT('',(0.00190441615676979,0.001,-0.00610189696988579));
#48385=CARTESIAN_POINT('',(0.00264938241039218,0.001,-0.00511483151597876));
#48386=CARTESIAN_POINT('',(0.00268708494896553,0.001,-0.00506487640301974));
#48387=CARTESIAN_POINT('',(0.00257866842927369,0.001,-0.00497627854900125));
#48388=CARTESIAN_POINT('',(0.00255021743138166,0.001,-0.00492053327615618));
#48389=CARTESIAN_POINT('',(0.00142633986350131,0.001,-0.00499880990860565));
#48390=CARTESIAN_POINT('',(0.00140969806589131,0.001,-0.00499913530392913));
#48391=CARTESIAN_POINT('',(0.00136135642578156,0.001,-0.00498929501065195));
#48392=CARTESIAN_POINT('Origin',(0.00142243003179848,0.001,-0.00479884812921755));
#48393=CARTESIAN_POINT('',(-0.00848709681638249,0.001,-0.00183103613732295));
#48394=CARTESIAN_POINT('',(-0.0084990215765556,0.001,-0.00182721203634963));
#48395=CARTESIAN_POINT('',(-0.00853149850581388,0.001,-0.00181051559890248));
#48396=CARTESIAN_POINT('Origin',(-0.00842602321036556,0.001,-0.00164058925588855));
#48397=CARTESIAN_POINT('',(-0.00804781744366059,0.001,-0.00368315161531047));
#48398=CARTESIAN_POINT('Origin',(-0.00926982557395217,0.001,-0.003));
#48399=CARTESIAN_POINT('',(-0.00778675335060335,0.001,-0.00360041384088911));
#48400=CARTESIAN_POINT('Origin',(-0.00787324485361894,0.001,-0.00378074470321196));
#48401=CARTESIAN_POINT('',(4.52079337441885E-5,0.001,-0.00735683187337398));
#48402=CARTESIAN_POINT('',(5.18147787824802E-5,0.001,-0.00736000069289933));
#48403=CARTESIAN_POINT('',(0.00400212262074066,0.001,-0.00858487618139458));
#48404=CARTESIAN_POINT('',(0.00409095201815433,0.001,-0.00861244474036231));
#48405=CARTESIAN_POINT('',(0.00439463505993757,0.001,-0.00758282450818601));
#48406=CARTESIAN_POINT('',(0.00441746175792763,0.001,-0.00752454984315485));
#48407=CARTESIAN_POINT('',(0.00428916220193663,0.001,-0.00746848786485146));
#48408=CARTESIAN_POINT('',(0.00424672634960324,0.001,-0.0074224857653085));
#48409=CARTESIAN_POINT('',(0.00310513229246118,0.001,-0.00782534372202691));
#48410=CARTESIAN_POINT('',(0.00316970710931718,0.001,-0.00780588145892302));
#48411=CARTESIAN_POINT('',(0.00283397885998211,0.001,-0.00748782871937848));
#48412=CARTESIAN_POINT('',(0.00287621909532571,0.001,-0.00754040674877505));
#48413=CARTESIAN_POINT('',(0.00343760106241995,0.001,-0.00640851728792926));
#48414=CARTESIAN_POINT('',(0.00346815021717762,0.001,-0.00635389363124816));
#48415=CARTESIAN_POINT('',(0.00334867942190192,0.001,-0.00628088369661617));
#48416=CARTESIAN_POINT('',(0.0033129027711333,0.001,-0.006229531715297));
#48417=CARTESIAN_POINT('',(0.00212708576461598,0.001,-0.00647319039387763));
#48418=CARTESIAN_POINT('',(0.00219370923929376,0.001,-0.00646270233976982));
#48419=CARTESIAN_POINT('',(0.00193910359020296,0.001,-0.00615973699598304));
#48420=CARTESIAN_POINT('',(-0.00926982557395217,0.001,-0.0024));
#48421=CARTESIAN_POINT('Origin',(-0.00926982557395217,0.001,-0.003));
#48422=CARTESIAN_POINT('Origin',(-0.00926982557395217,0.0172006855706717,
-0.003));
#48423=CARTESIAN_POINT('',(-0.00926982557395217,0.0129,-0.0025));
#48424=CARTESIAN_POINT('',(-0.00926982557395217,0.0129,-0.0035));
#48425=CARTESIAN_POINT('Origin',(-0.00926982557395217,0.0129,-0.003));
#48426=CARTESIAN_POINT('Origin',(-0.00926982557395217,0.0129,-0.003));
#48427=CARTESIAN_POINT('',(-0.00926982557395217,0.0011,-0.0025));
#48428=CARTESIAN_POINT('',(-0.00926982557395217,0.0172006855706717,-0.0025));
#48429=CARTESIAN_POINT('Origin',(-0.00926982557395217,0.0011,-0.003));
#48430=CARTESIAN_POINT('Origin',(0.00441815830616679,0.0011,-0.00465522418821883));
#48431=CARTESIAN_POINT('Origin',(0.00343760106241995,0.0011,-0.00640851728792926));
#48432=CARTESIAN_POINT('Origin',(0.00283397885998212,0.0011,-0.00748782871937848));
#48433=CARTESIAN_POINT('Origin',(-0.00703448893161721,0.0011,0.00479582892185301));
#48434=CARTESIAN_POINT('Origin',(0.00310513229246118,0.0011,-0.00782534372202691));
#48435=CARTESIAN_POINT('Origin',(0.00287621909532571,0.0129,-0.00754040674877505));
#48436=CARTESIAN_POINT('Origin',(0.00310513229246118,0.0129,-0.00782534372202691));
#48437=CARTESIAN_POINT('Origin',(0.00283397885998211,0.0129,-0.00748782871937848));
#48438=CARTESIAN_POINT('Origin',(0.00346815021717762,0.0129,-0.00635389363124816));
#48439=CARTESIAN_POINT('Origin',(0.00343760106241995,0.0129,-0.00640851728792926));
#48440=CARTESIAN_POINT('Origin',(-0.00512775505089191,0.0011,0.00588575838274743));
#48441=CARTESIAN_POINT('Origin',(0.00334867942190192,0.0011,-0.00628088369661617));
#48442=CARTESIAN_POINT('Origin',(-0.00524836317811532,0.0011,-0.0103430113609166));
#48443=CARTESIAN_POINT('Origin',(0.00428916220193663,0.0011,-0.00746848786485146));
#48444=CARTESIAN_POINT('Origin',(0.00316970710931718,0.0129,-0.00780588145892302));
#48445=CARTESIAN_POINT('Origin',(0.00428916220193663,0.0129,-0.00746848786485147));
#48446=CARTESIAN_POINT('Origin',(0.00331290277113331,0.0129,-0.006229531715297));
#48447=CARTESIAN_POINT('Origin',(0.00334867942190192,0.0129,-0.00628088369661617));
#48448=CARTESIAN_POINT('Origin',(-0.00753898540761223,0.0011,-0.00799485040867771));
#48449=CARTESIAN_POINT('Origin',(0.00212708576461597,0.0011,-0.00647319039387763));
#48450=CARTESIAN_POINT('Origin',(-0.00716170400106153,0.0011,0.00494469245223184));
#48451=CARTESIAN_POINT('Origin',(0.00439463505993757,0.0011,-0.00758282450818601));
#48452=CARTESIAN_POINT('Origin',(0.00424672634960323,0.0129,-0.00742248576530849));
#48453=CARTESIAN_POINT('Origin',(0.00439463505993757,0.0129,-0.00758282450818601));
#48454=CARTESIAN_POINT('Origin',(0.00219370923929376,0.0129,-0.00646270233976982));
#48455=CARTESIAN_POINT('Origin',(0.00212708576461598,0.0129,-0.00647319039387763));
#48456=CARTESIAN_POINT('Origin',(-0.00506603229059289,0.0011,0.00552107077956914));
#48457=CARTESIAN_POINT('Origin',(0.00190441615676979,0.0011,-0.00610189696988579));
#48458=CARTESIAN_POINT('Origin',(0.00617086596586019,0.0011,-0.00304825445754962));
#48459=CARTESIAN_POINT('Origin',(0.00400212262074066,0.0011,-0.00858487618139458));
#48460=CARTESIAN_POINT('Origin',(0.00441746175792763,0.0129,-0.00752454984315485));
#48461=CARTESIAN_POINT('Origin',(0.00400212262074066,0.0129,-0.00858487618139458));
#48462=CARTESIAN_POINT('Origin',(0.00193910359020296,0.0129,-0.00615973699598304));
#48463=CARTESIAN_POINT('Origin',(0.00190441615676979,0.0129,-0.00610189696988579));
#48464=CARTESIAN_POINT('Origin',(0.00222579787364439,0.0011,-0.00567607259367848));
#48465=CARTESIAN_POINT('Origin',(0.00264938241039218,0.0011,-0.00511483151597876));
#48466=CARTESIAN_POINT('Origin',(-0.0113833186128506,0.0011,-0.00380994292458512));
#48467=CARTESIAN_POINT('Origin',(4.52079337442121E-5,0.0011,-0.00735683187337399));
#48468=CARTESIAN_POINT('Origin',(4.52079337442124E-5,-0.0158951219150417,
-0.00735683187337399));
#48469=CARTESIAN_POINT('Origin',(4.52079337442121E-5,0.0129,-0.00735683187337399));
#48470=CARTESIAN_POINT('Origin',(4.52079337442123E-5,0.0011,-0.00735683187337399));
#48471=CARTESIAN_POINT('Origin',(0.00409095201815432,0.0129,-0.00861244474036231));
#48472=CARTESIAN_POINT('Origin',(4.52079337442158E-5,0.0129,-0.00735683187337399));
#48473=CARTESIAN_POINT('Origin',(0.00268708494896553,0.0129,-0.00506487640301974));
#48474=CARTESIAN_POINT('Origin',(0.00264938241039218,0.0129,-0.00511483151597876));
#48475=CARTESIAN_POINT('Origin',(-0.00309949089713811,0.0011,0.00614918503262233));
#48476=CARTESIAN_POINT('Origin',(0.00257866842927369,0.0011,-0.00497627854900125));
#48477=CARTESIAN_POINT('Origin',(4.52079337442135E-5,0.0011,-0.00735683187337399));
#48478=CARTESIAN_POINT('Origin',(4.52079337441885E-5,0.0011,-0.00735683187337398));
#48479=CARTESIAN_POINT('Origin',(4.52079337442119E-5,0.0129,-0.00735683187337399));
#48480=CARTESIAN_POINT('Origin',(4.52079337442122E-5,0.0129,-0.00735683187337399));
#48481=CARTESIAN_POINT('Origin',(0.00255021743138166,0.0129,-0.00492053327615618));
#48482=CARTESIAN_POINT('Origin',(0.00257866842927369,0.0129,-0.00497627854900125));
#48483=CARTESIAN_POINT('Origin',(-0.00910939770465845,0.0011,-0.00520481408041643));
#48484=CARTESIAN_POINT('Origin',(0.00142633986350131,0.0011,-0.00499880990860565));
#48485=CARTESIAN_POINT('Origin',(-0.0115661429208045,0.0011,-0.00178771755475424));
#48486=CARTESIAN_POINT('Origin',(-0.00778675335060335,0.0011,-0.00360041384088911));
#48487=CARTESIAN_POINT('Origin',(-0.00787324485361894,-0.0158951219150417,
-0.00378074470321196));
#48488=CARTESIAN_POINT('Origin',(-0.00787324485361894,0.0129,-0.00378074470321196));
#48489=CARTESIAN_POINT('Origin',(-0.00787324485361894,0.0011,-0.00378074470321196));
#48490=CARTESIAN_POINT('Origin',(5.18147787824767E-5,0.0129,-0.00736000069289933));
#48491=CARTESIAN_POINT('Origin',(-0.00778675335060335,0.0129,-0.00360041384088911));
#48492=CARTESIAN_POINT('Origin',(0.00140969806589131,0.0129,-0.00499913530392913));
#48493=CARTESIAN_POINT('Origin',(0.00142633986350131,0.0129,-0.00499880990860565));
#48494=CARTESIAN_POINT('Origin',(0.00142243003179848,-0.0158951219150417,
-0.00479884812921755));
#48495=CARTESIAN_POINT('Origin',(0.00142243003179848,0.0011,-0.00479884812921755));
#48496=CARTESIAN_POINT('Origin',(0.00142243003179848,0.0129,-0.00479884812921755));
#48497=CARTESIAN_POINT('Origin',(0.00142243003179848,0.0011,-0.00479884812921755));
#48498=CARTESIAN_POINT('Origin',(0.00136135642578156,0.0011,-0.00498929501065196));
#48499=CARTESIAN_POINT('Origin',(-0.00787324485361894,0.0011,-0.00378074470321196));
#48500=CARTESIAN_POINT('Origin',(-0.00804781744366059,0.0011,-0.00368315161531047));
#48501=CARTESIAN_POINT('Origin',(-0.00787324485361894,0.0129,-0.00378074470321196));
#48502=CARTESIAN_POINT('Origin',(-0.00804781744366059,0.0129,-0.00368315161531047));
#48503=CARTESIAN_POINT('Origin',(0.00142243003179848,0.0129,-0.00479884812921755));
#48504=CARTESIAN_POINT('Origin',(0.00136135642578156,0.0129,-0.00498929501065195));
#48505=CARTESIAN_POINT('Origin',(-0.0106016144887901,0.0011,-0.0011529403960444));
#48506=CARTESIAN_POINT('Origin',(-0.00848709681638249,0.0011,-0.00183103613732295));
#48507=CARTESIAN_POINT('Origin',(-0.00926982557395217,0.0011,-0.003));
#48508=CARTESIAN_POINT('Origin',(-0.00853149850581388,0.0011,-0.00181051559890248));
#48509=CARTESIAN_POINT('Origin',(-0.00926982557395217,0.0129,-0.003));
#48510=CARTESIAN_POINT('Origin',(-0.00853149850581388,0.0129,-0.00181051559890248));
#48511=CARTESIAN_POINT('Origin',(-0.0084990215765556,0.0129,-0.00182721203634963));
#48512=CARTESIAN_POINT('Origin',(-0.00848709681638249,0.0129,-0.00183103613732295));
#48513=CARTESIAN_POINT('Origin',(-0.00842602321036556,0.0011,-0.00164058925588855));
#48514=CARTESIAN_POINT('Origin',(-0.00842602321036556,0.0011,-0.00164058925588855));
#48515=CARTESIAN_POINT('Origin',(-0.00842602321036556,0.0129,-0.00164058925588855));
#48516=CARTESIAN_POINT('Origin',(-0.00842602321036556,0.0129,-0.00164058925588855));
#48517=CARTESIAN_POINT('Origin',(-0.00842602321036556,-0.0158951219150417,
-0.00164058925588855));
#48518=CARTESIAN_POINT('Origin',(-0.00926982557395217,0.0011,-0.003));
#48519=CARTESIAN_POINT('Origin',(-0.00926982557395217,0.0011,-0.0024));
#48520=CARTESIAN_POINT('Origin',(-0.00926982557395217,0.0129,-0.003));
#48521=CARTESIAN_POINT('Origin',(-0.00926982557395217,0.0129,-0.0036));
#54556=UNCERTAINTY_MEASURE_WITH_UNIT(LENGTH_MEASURE(1.E-5),#54581,
'DISTANCE_ACCURACY_VALUE',
'Maximum model space distance between geometric entities at asserted c
onnectivities');
#54564=UNCERTAINTY_MEASURE_WITH_UNIT(LENGTH_MEASURE(1.E-5),#54581,
'DISTANCE_ACCURACY_VALUE',
'Maximum model space distance between geometric entities at asserted c
onnectivities');
#54572=(
GEOMETRIC_REPRESENTATION_CONTEXT(3)
GLOBAL_UNCERTAINTY_ASSIGNED_CONTEXT((#54556))
GLOBAL_UNIT_ASSIGNED_CONTEXT((#54581,#54582,#54583))
REPRESENTATION_CONTEXT('','3D')
);
#54580=(
GEOMETRIC_REPRESENTATION_CONTEXT(3)
GLOBAL_UNCERTAINTY_ASSIGNED_CONTEXT((#54564))
GLOBAL_UNIT_ASSIGNED_CONTEXT((#54581,#54582,#54583))
REPRESENTATION_CONTEXT('','3D')
);
#54581=(
LENGTH_UNIT()
NAMED_UNIT(*)
SI_UNIT($,.METRE.)
);
#54582=(
NAMED_UNIT(*)
PLANE_ANGLE_UNIT()
SI_UNIT($,.RADIAN.)
);
#54583=(
NAMED_UNIT(*)
SI_UNIT($,.STERADIAN.)
SOLID_ANGLE_UNIT()
);
#54591=SHAPE_DEFINITION_REPRESENTATION(#54606,#54636);
#54606=PRODUCT_DEFINITION_SHAPE('',$,#54652);
#54636=SHAPE_REPRESENTATION('',(#18922),#54572);
#54644=PRODUCT_DEFINITION_CONTEXT('part definition',#54691,'design');
#54652=PRODUCT_DEFINITION('Part_6','Part_6',#54667,#54644);
#54667=PRODUCT_DEFINITION_FORMATION('',$,#54700);
#54691=APPLICATION_CONTEXT(
'Core Data for Automotive Mechanical Design Process');
#54692=PRODUCT_CONTEXT('part definition',#54691,'mechanical');
#54700=PRODUCT('Part_6','Part_6','Part 1',(#54692));
#54717=PRESENTATION_STYLE_ASSIGNMENT((#54727));
#54727=SURFACE_STYLE_USAGE(.BOTH.,#54737);
#54737=SURFACE_SIDE_STYLE('',(#54747));
#54747=SURFACE_STYLE_FILL_AREA(#54757);
#54757=FILL_AREA_STYLE('Opaque(202,209,238)',(#54767));
#54767=FILL_AREA_STYLE_COLOUR('Opaque(202,209,238)',#54777);
#54777=COLOUR_RGB('Opaque(202,209,238)', 0.09019608, 0.27058824, 0.51372549);
ENDSEC;
END-ISO-10303-21;
